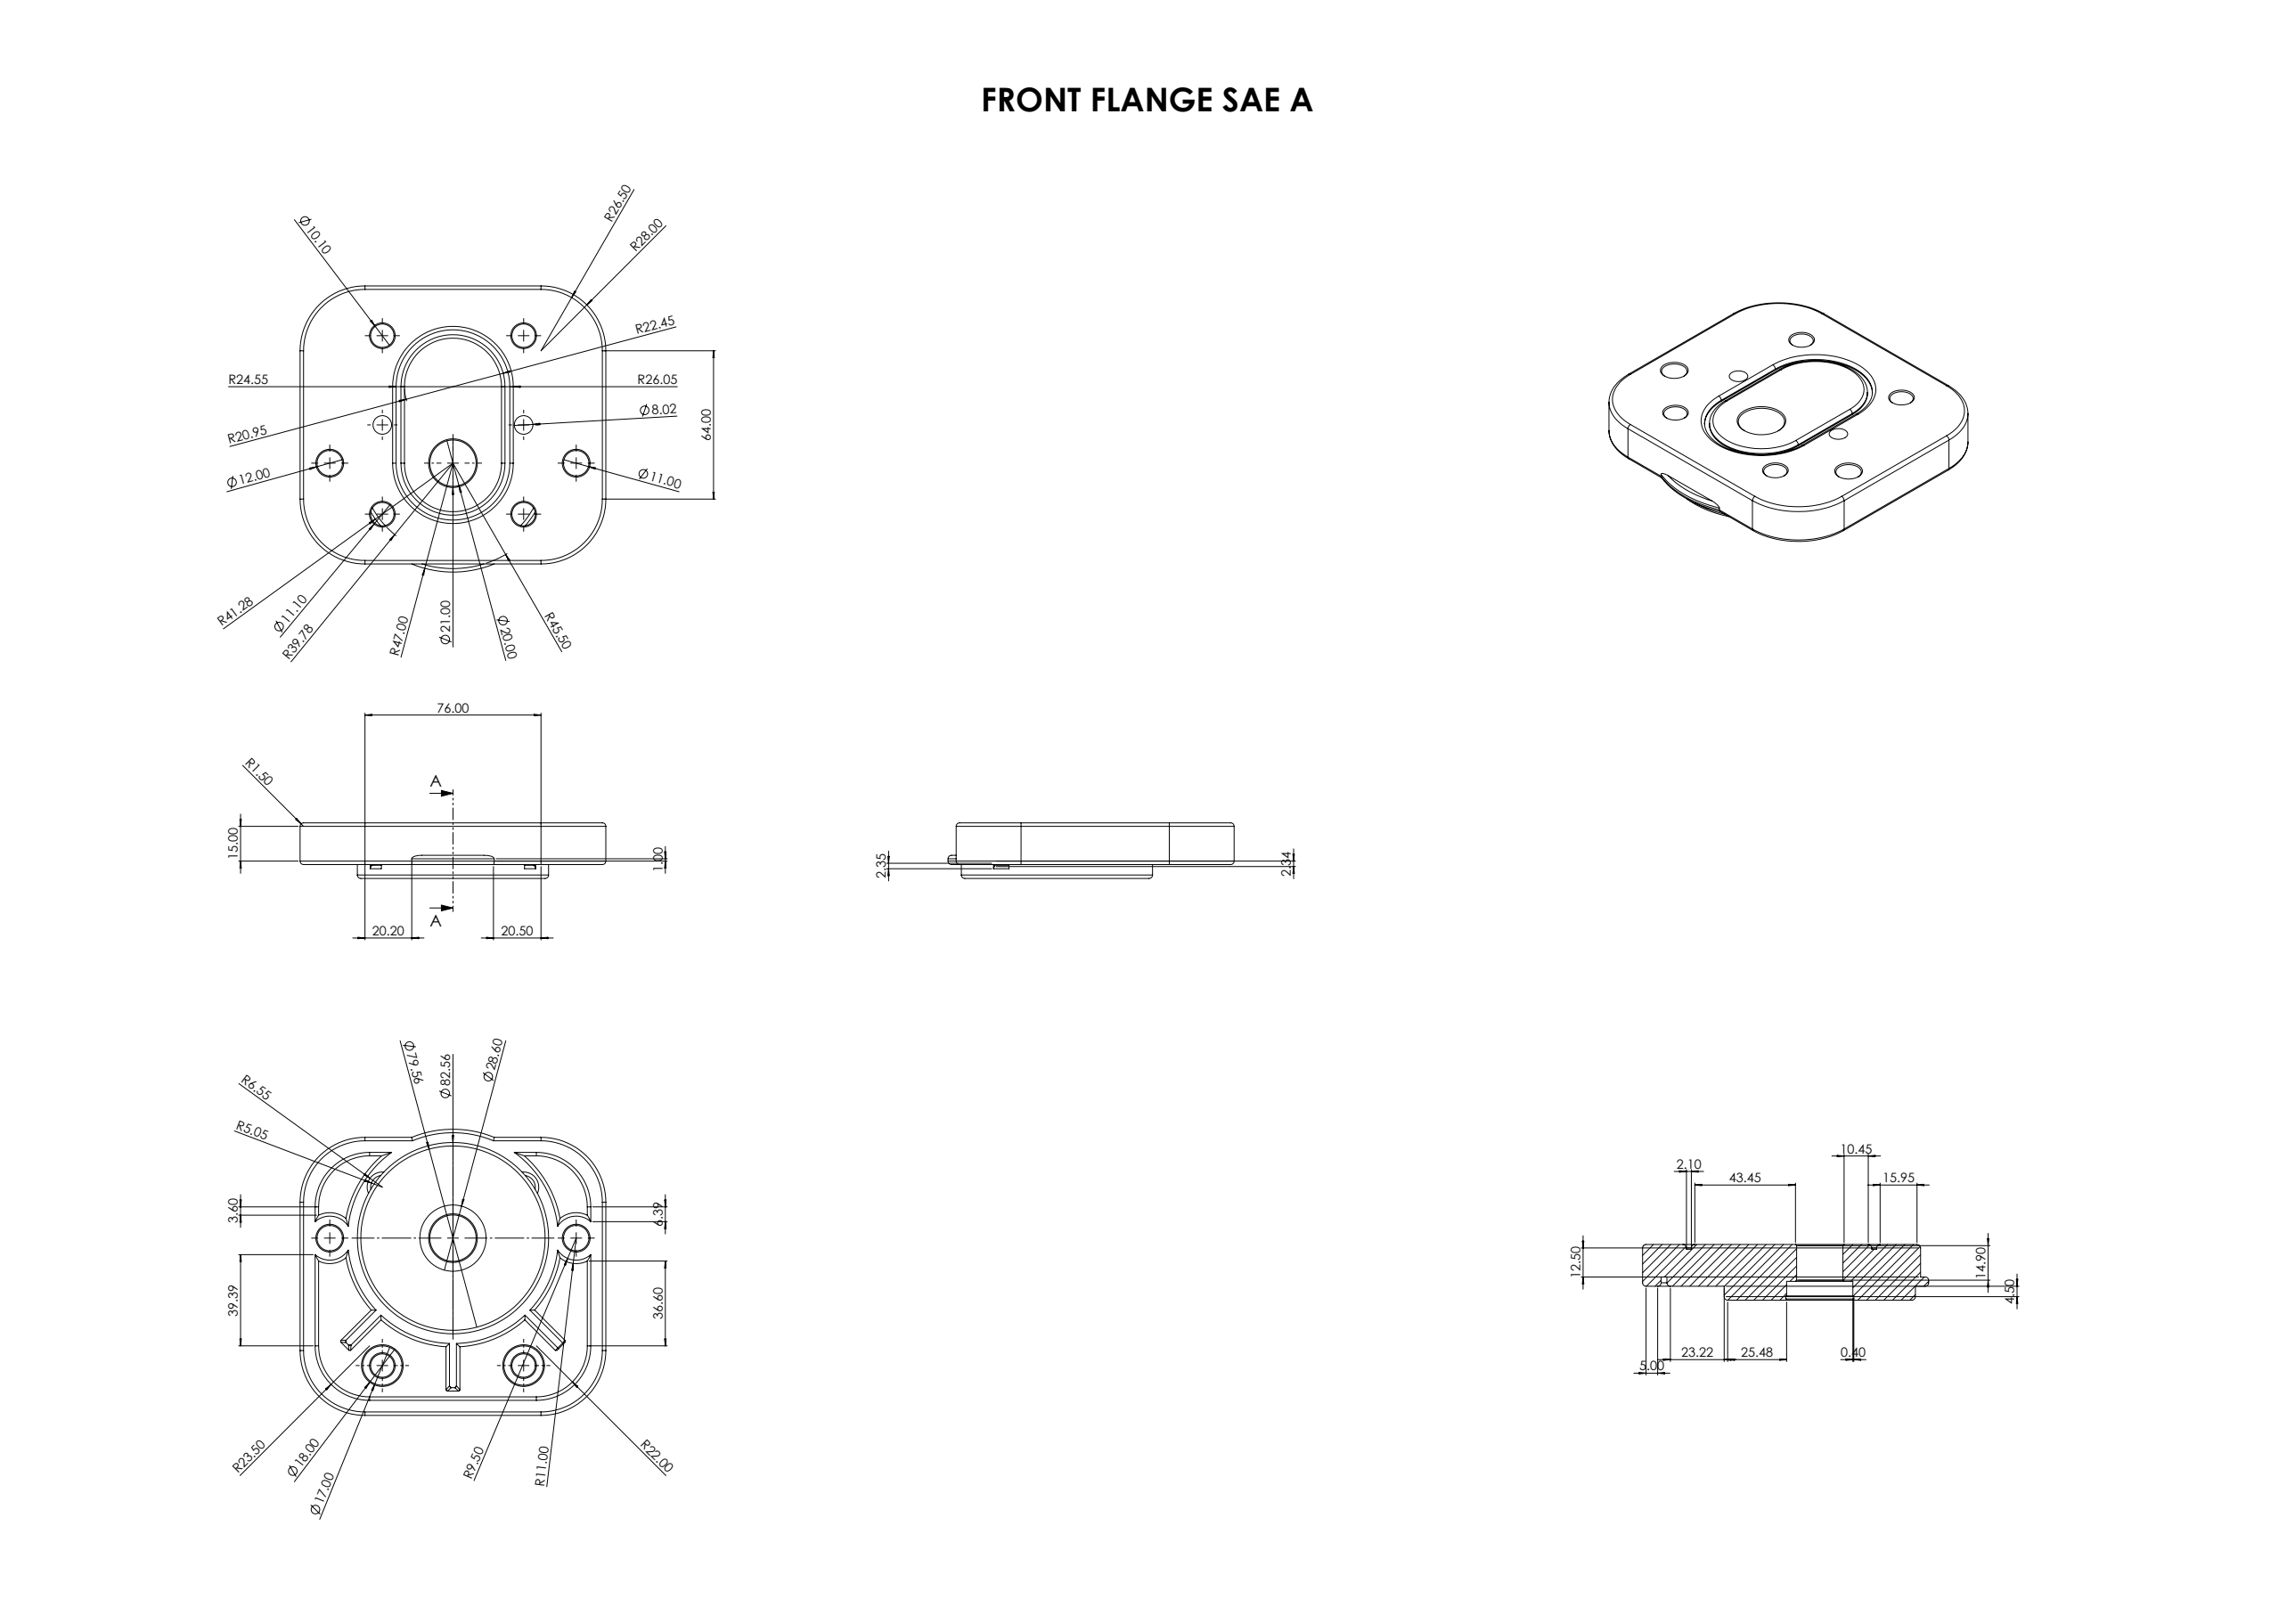
ISO-10303-21;
HEADER;
/* Generated by software containing ST-Developer
 * from STEP Tools, Inc. (www.steptools.com) 
 */

FILE_DESCRIPTION(
/* description */ (''),
/* implementation_level */ '2;1');

FILE_NAME(
/* name */ '01_Front_Flange_SAE_A.step',
/* time_stamp */ '2026-10-26T06:59:52-07:00',
/* author */ (''),
/* organization */ (''),
/* preprocessor_version */ 'ST-DEVELOPER v20.2',
/* originating_system */ 'Autodesk Translation Framework v15.15.0.0',
/* authorisation */ '');

FILE_SCHEMA (('AUTOMOTIVE_DESIGN { 1 0 10303 214 3 1 1 }'));
ENDSEC;

DATA;
#10=MECHANICAL_DESIGN_GEOMETRIC_PRESENTATION_REPRESENTATION('',(#164),#46395);
#136=SHAPE_REPRESENTATION_RELATIONSHIP('SRR','None',#46456,#150);
#150=ADVANCED_BREP_SHAPE_REPRESENTATION('',(#178),#46381);
#164=STYLED_ITEM('',(#46589),#178);
#178=MANIFOLD_SOLID_BREP('Body1',#24937);
#192=TOROIDAL_SURFACE('',#25235,45.5,1.5);
#193=TOROIDAL_SURFACE('',#25240,9.5,1.5);
#194=TOROIDAL_SURFACE('',#25242,45.5,1.5);
#195=TOROIDAL_SURFACE('',#25244,23.5,1.5);
#196=TOROIDAL_SURFACE('',#25255,45.5,1.5);
#197=TOROIDAL_SURFACE('',#25257,9.5,1.5);
#198=TOROIDAL_SURFACE('',#25259,23.5,1.5);
#199=TOROIDAL_SURFACE('',#25270,45.5,1.5);
#200=TOROIDAL_SURFACE('',#25271,45.5,1.5);
#201=TOROIDAL_SURFACE('',#25275,9.5,1.5);
#202=TOROIDAL_SURFACE('',#25281,9.5,1.5);
#203=TOROIDAL_SURFACE('',#25283,45.5,1.5);
#204=TOROIDAL_SURFACE('',#25285,23.5,1.5);
#205=TOROIDAL_SURFACE('',#25290,23.5,1.5);
#206=TOROIDAL_SURFACE('',#25308,26.5,1.5);
#207=TOROIDAL_SURFACE('',#25313,26.5,1.5);
#208=TOROIDAL_SURFACE('',#25318,26.5,1.5);
#209=TOROIDAL_SURFACE('',#25322,26.5,1.5);
#210=TOROIDAL_SURFACE('',#25338,45.5,1.5);
#211=TOROIDAL_SURFACE('',#25341,45.5,1.5);
#212=TOROIDAL_SURFACE('',#25348,26.5,1.5);
#213=TOROIDAL_SURFACE('',#25353,26.5,1.5);
#214=TOROIDAL_SURFACE('',#25357,26.5,1.5);
#215=TOROIDAL_SURFACE('',#25361,26.5,1.5);
#216=TOROIDAL_SURFACE('',#25365,39.78,1.5);
#217=TOROIDAL_SURFACE('',#25376,6.55,1.5);
#218=TOROIDAL_SURFACE('',#25377,39.78,1.5);
#219=TOROIDAL_SURFACE('',#25380,6.55,1.5);
#220=TOROIDAL_SURFACE('',#25381,39.78,1.5);
#221=TOROIDAL_SURFACE('',#25387,26.05,1.5);
#222=TOROIDAL_SURFACE('',#25392,26.05,1.5);
#223=TOROIDAL_SURFACE('',#25400,20.95,1.5);
#224=TOROIDAL_SURFACE('',#25405,20.95,1.5);
#235=B_SPLINE_CURVE_WITH_KNOTS('',3,(#33538,#33539,#33540,#33541,#33542,
#33543,#33544,#33545,#33546,#33547,#33548,#33549,#33550,#33551,#33552,#33553,
#33554,#33555,#33556,#33557,#33558,#33559,#33560,#33561,#33562,#33563,#33564,
#33565,#33566,#33567,#33568,#33569,#33570,#33571,#33572,#33573,#33574,#33575,
#33576,#33577,#33578,#33579,#33580,#33581,#33582,#33583,#33584,#33585,#33586,
#33587,#33588,#33589,#33590,#33591,#33592),.UNSPECIFIED.,.F.,.F.,(4,3,3,
3,3,3,3,3,3,3,3,3,3,3,3,3,3,3,4),(0.,0.0454718630237578,0.0931953780608733,
0.144039899823244,0.200168007589431,0.270586701890984,0.345292422598273,
0.401891619290293,0.45296463277568,0.503347839954974,0.552485563142507,
0.605298848839098,0.665634056697671,0.749225542523253,0.81191915689244,
0.864445081090996,0.913828865900519,0.959856605633726,1.),.UNSPECIFIED.);
#236=B_SPLINE_CURVE_WITH_KNOTS('',3,(#33594,#33595,#33596,#33597),
 .UNSPECIFIED.,.F.,.F.,(4,4),(0.,1.),.UNSPECIFIED.);
#237=B_SPLINE_CURVE_WITH_KNOTS('',3,(#33599,#33600,#33601,#33602,#33603,
#33604,#33605,#33606,#33607,#33608,#33609,#33610,#33611,#33612,#33613,#33614,
#33615,#33616,#33617,#33618,#33619,#33620,#33621,#33622,#33623,#33624,#33625,
#33626,#33627,#33628,#33629,#33630,#33631,#33632,#33633,#33634,#33635,#33636,
#33637,#33638,#33639,#33640,#33641,#33642,#33643,#33644,#33645,#33646,#33647,
#33648,#33649,#33650,#33651,#33652,#33653),.UNSPECIFIED.,.F.,.F.,(4,3,3,
3,3,3,3,3,3,3,3,3,3,3,3,3,3,3,4),(0.,0.0454743571758902,0.0932006890496271,
0.144048574957132,0.200181673047708,0.270614812390332,0.345307027643268,
0.401906381576284,0.452980318796508,0.503379519506553,0.552517196305264,
0.605331277143632,0.665671120969931,0.749253340727448,0.811940005545586,
0.864461351673364,0.913841478931635,0.959866376898225,1.),.UNSPECIFIED.);
#238=B_SPLINE_CURVE_WITH_KNOTS('',3,(#33680,#33681,#33682,#33683,#33684,
#33685),.UNSPECIFIED.,.F.,.F.,(4,1,1,4),(-1.75610615531805,-1.00348923161032,
-0.501744615805158,5.55111512312578E-16),.UNSPECIFIED.);
#239=B_SPLINE_CURVE_WITH_KNOTS('',3,(#33688,#33689,#33690,#33691,#33692,
#33693),.UNSPECIFIED.,.F.,.F.,(4,1,1,4),(-5.55111512312578E-16,0.501744615805158,
1.00348923161032,1.75610615531805),.UNSPECIFIED.);
#240=B_SPLINE_CURVE_WITH_KNOTS('',3,(#33804,#33805,#33806,#33807,#33808,
#33809,#33810),.UNSPECIFIED.,.F.,.F.,(4,1,1,1,4),(-1.75610615531805,-1.25436153951289,
-0.752616923707736,-0.501744615805158,1.11022302462516E-16),
 .UNSPECIFIED.);
#241=B_SPLINE_CURVE_WITH_KNOTS('',3,(#33811,#33812,#33813,#33814,#33815,
#33816,#33817,#33818,#33819,#33820,#33821,#33822,#33823,#33824,#33825,#33826,
#33827,#33828,#33829,#33830,#33831,#33832,#33833,#33834,#33835,#33836,#33837,
#33838,#33839,#33840,#33841,#33842,#33843,#33844,#33845,#33846,#33847,#33848,
#33849,#33850,#33851,#33852,#33853,#33854,#33855,#33856,#33857,#33858,#33859,
#33860,#33861,#33862,#33863,#33864,#33865),.UNSPECIFIED.,.F.,.F.,(4,3,3,
3,3,3,3,3,3,3,3,3,3,3,3,3,3,3,4),(0.,0.0454718630243312,0.0931953780626333,
0.144039899827111,0.200168007593285,0.270586701897688,0.345292422601244,
0.401891619293199,0.452964632777224,0.503347839955881,0.552485563143915,
0.605298848838407,0.665634056695417,0.749225542521563,0.811919156891172,
0.864445081089317,0.913828865898997,0.959856605632299,1.),.UNSPECIFIED.);
#242=B_SPLINE_CURVE_WITH_KNOTS('',3,(#33895,#33896,#33897,#33898),
 .UNSPECIFIED.,.F.,.F.,(4,4),(0.,1.),.UNSPECIFIED.);
#243=B_SPLINE_CURVE_WITH_KNOTS('',3,(#33899,#33900,#33901,#33902,#33903,
#33904,#33905,#33906,#33907,#33908,#33909,#33910,#33911,#33912,#33913,#33914,
#33915,#33916,#33917,#33918,#33919,#33920,#33921,#33922,#33923,#33924,#33925,
#33926,#33927,#33928,#33929,#33930,#33931,#33932,#33933,#33934,#33935,#33936,
#33937,#33938,#33939,#33940,#33941,#33942,#33943,#33944,#33945,#33946,#33947,
#33948,#33949,#33950,#33951,#33952,#33953),.UNSPECIFIED.,.F.,.F.,(4,3,3,
3,3,3,3,3,3,3,3,3,3,3,3,3,3,3,4),(0.,0.0454743571758495,0.0932006890494206,
0.144048574957566,0.200181673048685,0.270614812390706,0.345307027641822,
0.401906381575635,0.452980318795634,0.503379519504597,0.552517196303257,
0.605331277141522,0.665671120968433,0.749253340726325,0.811940005544743,
0.864461351672607,0.913841478930594,0.959866376897371,1.),.UNSPECIFIED.);
#244=B_SPLINE_CURVE_WITH_KNOTS('',3,(#33984,#33985,#33986,#33987,#33988,
#33989,#33990),.UNSPECIFIED.,.F.,.F.,(4,1,1,1,4),(-1.11022302462516E-16,
0.501744615805158,0.752616923707736,1.25436153951289,1.75610615531805),
 .UNSPECIFIED.);
#245=B_SPLINE_CURVE_WITH_KNOTS('',3,(#33998,#33999,#34000,#34001,#34002,
#34003,#34004,#34005,#34006,#34007,#34008,#34009,#34010,#34011),
 .UNSPECIFIED.,.F.,.F.,(4,2,2,2,2,2,4),(0.2830029806958,0.32673657269417,
0.376100941370913,0.440377410457652,0.50187293467793,0.56600596139079,0.566744275786352),
 .UNSPECIFIED.);
#246=B_SPLINE_CURVE_WITH_KNOTS('',3,(#34035,#34036,#34037,#34038,#34039,
#34040),.UNSPECIFIED.,.F.,.F.,(4,2,4),(0.457345926229208,0.511458202087047,
0.555227226239397),.UNSPECIFIED.);
#247=B_SPLINE_CURVE_WITH_KNOTS('',3,(#34044,#34045,#34046,#34047,#34048,
#34049),.UNSPECIFIED.,.F.,.F.,(4,2,4),(0.,0.0542493992714901,0.0984920623079337),
 .UNSPECIFIED.);
#248=B_SPLINE_CURVE_WITH_KNOTS('',3,(#34058,#34059,#34060,#34061,#34062,
#34063,#34064,#34065),.UNSPECIFIED.,.F.,.F.,(4,2,2,4),(0.,0.0729822624604683,
0.159547666524593,0.160512003570787),.UNSPECIFIED.);
#249=B_SPLINE_CURVE_WITH_KNOTS('',3,(#34071,#34072,#34073,#34074,#34075,
#34076,#34077,#34078),.UNSPECIFIED.,.F.,.F.,(4,2,2,4),(0.883241961717341,
0.890937005468247,0.9697019851369,1.04402990736473),.UNSPECIFIED.);
#250=B_SPLINE_CURVE_WITH_KNOTS('',3,(#34083,#34084,#34085,#34086,#34087,
#34088),.UNSPECIFIED.,.F.,.F.,(4,2,4),(-0.0984920602555225,-0.0542493992714899,
0.),.UNSPECIFIED.);
#251=B_SPLINE_CURVE_WITH_KNOTS('',3,(#34092,#34093,#34094,#34095,#34096,
#34097),.UNSPECIFIED.,.F.,.F.,(4,2,4),(0.359464626219636,0.403233650371369,
0.457345926229208),.UNSPECIFIED.);
#252=B_SPLINE_CURVE_WITH_KNOTS('',3,(#34106,#34107,#34108,#34109,#34110,
#34111,#34112,#34113),.UNSPECIFIED.,.F.,.F.,(4,2,2,4),(0.883254863276601,
0.890921572363312,0.969698219486375,1.04404196291709),.UNSPECIFIED.);
#253=B_SPLINE_CURVE_WITH_KNOTS('',3,(#34117,#34118,#34119,#34120,#34121,
#34122,#34123,#34124),.UNSPECIFIED.,.F.,.F.,(4,2,2,4),(0.,0.0729893210250683,
0.159554275962458,0.160511436887519),.UNSPECIFIED.);
#254=B_SPLINE_CURVE_WITH_KNOTS('',3,(#34130,#34131,#34132,#34133,#34134,
#34135),.UNSPECIFIED.,.F.,.F.,(4,2,4),(0.457345926229207,0.511458202087047,
0.555227226239396),.UNSPECIFIED.);
#255=B_SPLINE_CURVE_WITH_KNOTS('',3,(#34137,#34138,#34139,#34140,#34141,
#34142),.UNSPECIFIED.,.F.,.F.,(4,2,4),(0.,0.0542493992714896,0.0984920622777539),
 .UNSPECIFIED.);
#256=B_SPLINE_CURVE_WITH_KNOTS('',3,(#34146,#34147,#34148,#34149,#34150,
#34151),.UNSPECIFIED.,.F.,.F.,(4,2,4),(-0.0984920602555227,-0.0542493992714901,
0.),.UNSPECIFIED.);
#257=B_SPLINE_CURVE_WITH_KNOTS('',3,(#34153,#34154,#34155,#34156,#34157,
#34158),.UNSPECIFIED.,.F.,.F.,(4,2,4),(0.359464626219636,0.403233650371367,
0.457345926229207),.UNSPECIFIED.);
#258=B_SPLINE_CURVE_WITH_KNOTS('',3,(#34250,#34251,#34252,#34253,#34254,
#34255,#34256,#34257,#34258,#34259,#34260,#34261,#34262,#34263,#34264,#34265,
#34266,#34267,#34268,#34269,#34270,#34271,#34272,#34273,#34274,#34275,#34276,
#34277,#34278,#34279,#34280,#34281,#34282,#34283,#34284,#34285,#34286,#34287,
#34288,#34289,#34290,#34291,#34292,#34293,#34294,#34295,#34296,#34297,#34298,
#34299,#34300,#34301,#34302,#34303,#34304),.UNSPECIFIED.,.F.,.F.,(4,3,3,
3,3,3,3,3,3,3,3,3,3,3,3,3,3,3,4),(0.,0.0454718630236453,0.0931953780618335,
0.144039899826865,0.200168007592162,0.270586701896513,0.345292422605783,
0.401891619297809,0.452964632782272,0.503347839964507,0.552485563152053,
0.605298848849878,0.665634056712773,0.74922554253458,0.811919156900935,
0.864445081098314,0.913828865908445,0.959856605641832,1.),.UNSPECIFIED.);
#259=B_SPLINE_CURVE_WITH_KNOTS('',3,(#34306,#34307,#34308,#34309),
 .UNSPECIFIED.,.F.,.F.,(4,4),(0.,1.),.UNSPECIFIED.);
#260=B_SPLINE_CURVE_WITH_KNOTS('',3,(#34310,#34311,#34312,#34313,#34314,
#34315,#34316,#34317,#34318,#34319,#34320,#34321,#34322,#34323,#34324,#34325,
#34326,#34327,#34328,#34329,#34330,#34331,#34332,#34333,#34334,#34335,#34336,
#34337,#34338,#34339,#34340,#34341,#34342,#34343,#34344,#34345,#34346,#34347,
#34348,#34349,#34350,#34351,#34352,#34353,#34354,#34355,#34356,#34357,#34358,
#34359,#34360,#34361,#34362,#34363,#34364),.UNSPECIFIED.,.F.,.F.,(4,3,3,
3,3,3,3,3,3,3,3,3,3,3,3,3,3,3,4),(0.,0.0454743571759648,0.0932006890496545,
0.144048574957612,0.200181673048621,0.270614812391917,0.345307027644055,
0.401906381576845,0.452980318797118,0.503379519507497,0.552517196306345,
0.605331277144942,0.665671120971507,0.74925334072863,0.811940005546473,
0.864461351674218,0.91384147893233,0.959866376898877,1.),.UNSPECIFIED.);
#261=B_SPLINE_CURVE_WITH_KNOTS('',3,(#34390,#34391,#34392,#34393,#34394,
#34395),.UNSPECIFIED.,.F.,.F.,(4,1,1,4),(-1.75610615531806,-1.00348923161031,
-0.501744615805142,2.47024622979097E-14),.UNSPECIFIED.);
#262=B_SPLINE_CURVE_WITH_KNOTS('',3,(#34398,#34399,#34400,#34401,#34402,
#34403),.UNSPECIFIED.,.F.,.F.,(4,1,1,4),(-2.47024622979097E-14,0.501744615805142,
1.00348923161031,1.75610615531806),.UNSPECIFIED.);
#263=B_SPLINE_CURVE_WITH_KNOTS('',3,(#34414,#34415,#34416,#34417,#34418,
#34419),.UNSPECIFIED.,.F.,.F.,(4,1,1,4),(-1.75610615531805,-1.00348923161031,
-0.501744615805157,-5.27355936696957E-16),.UNSPECIFIED.);
#264=B_SPLINE_CURVE_WITH_KNOTS('',3,(#34420,#34421,#34422,#34423,#34424,
#34425,#34426,#34427,#34428,#34429,#34430,#34431,#34432,#34433,#34434,#34435,
#34436,#34437,#34438,#34439,#34440,#34441,#34442,#34443,#34444,#34445,#34446,
#34447,#34448,#34449,#34450,#34451,#34452,#34453,#34454,#34455,#34456,#34457,
#34458,#34459,#34460,#34461,#34462,#34463,#34464,#34465,#34466,#34467,#34468,
#34469,#34470,#34471,#34472,#34473,#34474),.UNSPECIFIED.,.F.,.F.,(4,3,3,
3,3,3,3,3,3,3,3,3,3,3,3,3,3,3,4),(0.,0.0454718630243914,0.0931953780626216,
0.14403989982724,0.200168007593373,0.270586701897748,0.345292422601248,
0.401891619293078,0.452964632777054,0.50334783995564,0.552485563143574,
0.605298848838025,0.665634056695,0.74922554252125,0.811919156890937,0.864445081089107,
0.91382886589878,0.959856605632085,1.),.UNSPECIFIED.);
#265=B_SPLINE_CURVE_WITH_KNOTS('',3,(#34504,#34505,#34506,#34507),
 .UNSPECIFIED.,.F.,.F.,(4,4),(0.,1.),.UNSPECIFIED.);
#266=B_SPLINE_CURVE_WITH_KNOTS('',3,(#34508,#34509,#34510,#34511,#34512,
#34513,#34514,#34515,#34516,#34517,#34518,#34519,#34520,#34521,#34522,#34523,
#34524,#34525,#34526,#34527,#34528,#34529,#34530,#34531,#34532,#34533,#34534,
#34535,#34536,#34537,#34538,#34539,#34540,#34541,#34542,#34543,#34544,#34545,
#34546,#34547,#34548,#34549,#34550,#34551,#34552,#34553,#34554,#34555,#34556,
#34557,#34558,#34559,#34560,#34561,#34562),.UNSPECIFIED.,.F.,.F.,(4,3,3,
3,3,3,3,3,3,3,3,3,3,3,3,3,3,3,4),(0.,0.0454743571761675,0.0932006890500933,
0.144048574956671,0.200181673048282,0.270614812391009,0.345307027645443,
0.401906381578876,0.452980318799016,0.503379519512151,0.552517196310239,
0.605331277149278,0.665671120975839,0.749253340731879,0.81194000554891,
0.864461351676132,0.91384147893387,0.959866376900601,1.),.UNSPECIFIED.);
#267=B_SPLINE_CURVE_WITH_KNOTS('',3,(#34589,#34590,#34591,#34592,#34593,
#34594),.UNSPECIFIED.,.F.,.F.,(4,1,1,4),(5.27355936696957E-16,0.501744615805157,
1.00348923161031,1.75610615531805),.UNSPECIFIED.);
#268=B_SPLINE_CURVE_WITH_KNOTS('',3,(#34602,#34603,#34604,#34605,#34606,
#34607,#34608,#34609,#34610,#34611,#34612,#34613,#34614,#34615),
 .UNSPECIFIED.,.F.,.F.,(4,2,2,2,2,2,4),(-0.566727656910624,-0.565965930395602,
-0.501954114034259,-0.440929548119714,-0.376258061364955,-0.326742970835578,
-0.282982965197809),.UNSPECIFIED.);
#269=B_SPLINE_CURVE_WITH_KNOTS('',3,(#34659,#34660,#34661,#34662,#34663,
#34664,#34665,#34666,#34667,#34668,#34669,#34670),.UNSPECIFIED.,.F.,.F.,
(4,2,2,2,2,4),(0.,0.0177298768866499,0.0386480203638908,0.106699501354674,
0.29072652917135,0.474753556988026),.UNSPECIFIED.);
#270=B_SPLINE_CURVE_WITH_KNOTS('',3,(#34674,#34675,#34676,#34677,#34678,
#34679,#34680,#34681,#34682,#34683,#34684,#34685),.UNSPECIFIED.,.F.,.F.,
(4,2,2,2,2,4),(1.80681462537756,1.99084165319423,2.17486868101091,2.24292016200169,
2.26383830547893,2.28156818236558),.UNSPECIFIED.);
#271=B_SPLINE_CURVE_WITH_KNOTS('',3,(#34695,#34696,#34697,#34698,#34699,
#34700,#34701,#34702,#34703,#34704,#34705,#34706,#34707,#34708),
 .UNSPECIFIED.,.F.,.F.,(4,2,2,2,2,2,4),(-1.39612360577563,-1.39460700772923,
-1.17311194871629,-0.972537848487119,-0.846807900198276,-0.765057233826425,
-0.697303504183967),.UNSPECIFIED.);
#272=B_SPLINE_CURVE_WITH_KNOTS('',3,(#34711,#34712,#34713,#34714,#34715,
#34716,#34717,#34718,#34719,#34720,#34721,#34722,#34723,#34724),
 .UNSPECIFIED.,.F.,.F.,(4,2,2,2,2,2,4),(-0.00127041341091992,0.,0.142293631997042,
0.26745747621236,0.346088913132952,0.397847011808156,0.440929147841825),
 .UNSPECIFIED.);
#273=B_SPLINE_CURVE_WITH_KNOTS('',3,(#34727,#34728,#34729,#34730,#34731,
#34732,#34733,#34734,#34735,#34736,#34737,#34738,#34739,#34740),
 .UNSPECIFIED.,.F.,.F.,(4,2,2,2,2,2,4),(-1.41597302520629,-1.41418889589625,
-1.0666111176201,-0.892135751403682,-0.801536275589833,-0.748843387075389,
-0.707094447966972),.UNSPECIFIED.);
#274=B_SPLINE_CURVE_WITH_KNOTS('',3,(#34768,#34769,#34770,#34771,#34772,
#34773,#34774,#34775,#34776,#34777,#34778,#34779,#34780,#34781),
 .UNSPECIFIED.,.F.,.F.,(4,2,2,2,2,2,4),(-1.39362312416001,-1.39199898884262,
-1.17364167365164,-0.971197013124251,-0.845224951582453,-0.76357754542349,
-0.695999491978471),.UNSPECIFIED.);
#275=B_SPLINE_CURVE_WITH_KNOTS('',3,(#34784,#34785,#34786,#34787,#34788,
#34789,#34790,#34791,#34792,#34793,#34794,#34795,#34796,#34797),
 .UNSPECIFIED.,.F.,.F.,(4,2,2,2,2,2,4),(-0.00178412931182033,0.,0.347577778842949,
0.522053145574294,0.612652621655965,0.665345510326134,0.707094449558532),
 .UNSPECIFIED.);
#276=B_SPLINE_CURVE_WITH_KNOTS('',3,(#34800,#34801,#34802,#34803,#34804,
#34805,#34806,#34807,#34808,#34809,#34810,#34811,#34812,#34813),
 .UNSPECIFIED.,.F.,.F.,(4,2,2,2,2,2,4),(-0.883128709093834,-0.881858295682913,
-0.739564663685846,-0.614400819470615,-0.535769382550153,-0.484011283875034,
-0.440929147841436),.UNSPECIFIED.);
#277=B_SPLINE_CURVE_WITH_KNOTS('',3,(#34840,#34841,#34842,#34843,#34844,
#34845,#34846,#34847,#34848,#34849,#34850,#34851,#34852,#34853),
 .UNSPECIFIED.,.F.,.F.,(4,2,2,2,2,2,4),(0.237947781581816,0.295547529372161,
0.353697178748574,0.412988302648374,0.444419571172075,0.475895563163675,
0.476565408893143),.UNSPECIFIED.);
#278=B_SPLINE_CURVE_WITH_KNOTS('',3,(#34854,#34855,#34856,#34857,#34858,
#34859,#34860,#34861,#34862,#34863,#34864,#34865,#34866,#34867),
 .UNSPECIFIED.,.F.,.F.,(4,2,2,2,2,2,4),(-0.000669845729473591,0.,0.0314759919915142,
0.0629072605151251,0.122198384414748,0.180348033790988,0.237947781581162),
 .UNSPECIFIED.);
#279=B_SPLINE_CURVE_WITH_KNOTS('',3,(#34871,#34872,#34873,#34874,#34875,
#34876,#34877,#34878,#34879,#34880,#34881,#34882,#34883,#34884),
 .UNSPECIFIED.,.F.,.F.,(4,2,2,2,2,2,4),(-0.000737243235122344,0.,0.0641388256771107,
0.1256562494953,0.189914332907335,0.239271567314492,0.283003897177937),
 .UNSPECIFIED.);
#280=B_SPLINE_CURVE_WITH_KNOTS('',3,(#34891,#34892,#34893,#34894,#34895,
#34896,#34897,#34898,#34899,#34900,#34901,#34902,#34903,#34904),
 .UNSPECIFIED.,.F.,.F.,(4,2,2,2,2,2,4),(0.440929147841474,0.484011283875067,
0.53576938255019,0.614400819470681,0.739564663685834,0.881858295682709,
0.883128709093627),.UNSPECIFIED.);
#281=B_SPLINE_CURVE_WITH_KNOTS('',3,(#34907,#34908,#34909,#34910,#34911,
#34912,#34913,#34914,#34915,#34916,#34917,#34918,#34919,#34920),
 .UNSPECIFIED.,.F.,.F.,(4,2,2,2,2,2,4),(-0.00151659805374153,0.,0.221495058999754,
0.422069157956912,0.547799105448391,0.629549771301697,0.697303500514436),
 .UNSPECIFIED.);
#282=B_SPLINE_CURVE_WITH_KNOTS('',3,(#34932,#34933,#34934,#34935,#34936,
#34937,#34938,#34939,#34940,#34941,#34942,#34943,#34944,#34945),
 .UNSPECIFIED.,.F.,.F.,(4,2,2,2,2,2,4),(-0.00127041341147968,0.,0.142293632019536,
0.267457476256502,0.346088913190727,0.397847011874902,0.44092914791602),
 .UNSPECIFIED.);
#283=B_SPLINE_CURVE_WITH_KNOTS('',3,(#34948,#34949,#34950,#34951,#34952,
#34953,#34954,#34955,#34956,#34957,#34958,#34959,#34960,#34961),
 .UNSPECIFIED.,.F.,.F.,(4,2,2,2,2,2,4),(-1.39612359503373,-1.39460699698273,
-1.17311193853035,-0.972537840238686,-0.846807893164431,-0.765057227582403,
-0.697303498594505),.UNSPECIFIED.);
#284=B_SPLINE_CURVE_WITH_KNOTS('',3,(#34965,#34966,#34967,#34968,#34969,
#34970,#34971,#34972,#34973,#34974,#34975,#34976,#34977,#34978),
 .UNSPECIFIED.,.F.,.F.,(4,2,2,2,2,2,4),(0.283003897184326,0.326736227048831,
0.37609346145714,0.440351544870681,0.501868968690292,0.566007794368658,
0.566745037603787),.UNSPECIFIED.);
#285=B_SPLINE_CURVE_WITH_KNOTS('',3,(#35089,#35090,#35091,#35092,#35093,
#35094,#35095,#35096,#35097,#35098,#35099,#35100,#35101,#35102),
 .UNSPECIFIED.,.F.,.F.,(4,2,2,2,2,2,4),(-0.000738314395613078,0.,0.0641330267183371,
0.125628550943858,0.189905020036076,0.23926938871703,0.283002980719128),
 .UNSPECIFIED.);
#286=B_SPLINE_CURVE_WITH_KNOTS('',3,(#35105,#35106,#35107,#35108,#35109,
#35110,#35111,#35112,#35113,#35114,#35115,#35116,#35117,#35118),
 .UNSPECIFIED.,.F.,.F.,(4,2,2,2,2,2,4),(-0.000761726515024963,0.,0.0640118163614976,
0.125036382276213,0.189707869031154,0.239222959560681,0.282982965198561),
 .UNSPECIFIED.);
#287=B_SPLINE_CURVE_WITH_KNOTS('',3,(#35161,#35162,#35163,#35164,#35165,
#35166,#35167,#35168),.UNSPECIFIED.,.F.,.F.,(4,2,2,4),(0.9079700629405,
0.928682763365301,1.00209186414222,1.07647666313639),.UNSPECIFIED.);
#288=B_SPLINE_CURVE_WITH_KNOTS('',3,(#35169,#35170,#35171,#35172,#35173,
#35174),.UNSPECIFIED.,.F.,.F.,(4,2,4),(0.,0.0943434934286175,0.17124459577731),
 .UNSPECIFIED.);
#289=B_SPLINE_CURVE_WITH_KNOTS('',3,(#35176,#35177,#35178,#35179,#35180,
#35181,#35182,#35183),.UNSPECIFIED.,.F.,.F.,(4,2,2,4),(0.907970062940467,
0.928682763365269,1.00209186414218,1.07647666313636),.UNSPECIFIED.);
#290=B_SPLINE_CURVE_WITH_KNOTS('',3,(#35185,#35186,#35187,#35188,#35189,
#35190),.UNSPECIFIED.,.F.,.F.,(4,2,4),(0.,0.0943434934286164,0.171244595777307),
 .UNSPECIFIED.);
#390=B_SPLINE_SURFACE_WITH_KNOTS('',3,3,((#33512,#33513,#33514,#33515,#33516,
#33517),(#33518,#33519,#33520,#33521,#33522,#33523),(#33524,#33525,#33526,
#33527,#33528,#33529),(#33530,#33531,#33532,#33533,#33534,#33535)),
 .UNSPECIFIED.,.F.,.F.,.F.,(4,4),(4,1,1,4),(0.,1.),(0.,0.571428571428571,
0.857142857142857,1.),.UNSPECIFIED.);
#391=B_SPLINE_SURFACE_WITH_KNOTS('',3,3,((#33655,#33656,#33657,#33658,#33659,
#33660),(#33661,#33662,#33663,#33664,#33665,#33666),(#33667,#33668,#33669,
#33670,#33671,#33672),(#33673,#33674,#33675,#33676,#33677,#33678)),
 .UNSPECIFIED.,.F.,.F.,.F.,(4,4),(4,1,1,4),(0.,1.),(-1.75610615531805,-1.00348923161032,
-0.501744615805158,5.55111512312578E-16),.UNSPECIFIED.);
#392=B_SPLINE_SURFACE_WITH_KNOTS('',3,3,((#33870,#33871,#33872,#33873,#33874,
#33875),(#33876,#33877,#33878,#33879,#33880,#33881),(#33882,#33883,#33884,
#33885,#33886,#33887),(#33888,#33889,#33890,#33891,#33892,#33893)),
 .UNSPECIFIED.,.F.,.F.,.F.,(4,4),(4,1,1,4),(0.,1.),(0.,0.571428571428571,
0.857142857142857,1.),.UNSPECIFIED.);
#393=B_SPLINE_SURFACE_WITH_KNOTS('',3,3,((#33954,#33955,#33956,#33957,#33958,
#33959,#33960),(#33961,#33962,#33963,#33964,#33965,#33966,#33967),(#33968,
#33969,#33970,#33971,#33972,#33973,#33974),(#33975,#33976,#33977,#33978,
#33979,#33980,#33981)),.UNSPECIFIED.,.F.,.F.,.F.,(4,4),(4,1,1,1,4),(0.,
1.),(-1.75610615531805,-1.25436153951289,-0.752616923707736,-0.501744615805158,
1.11022302462516E-16),.UNSPECIFIED.);
#394=B_SPLINE_SURFACE_WITH_KNOTS('',3,3,((#34225,#34226,#34227,#34228,#34229,
#34230),(#34231,#34232,#34233,#34234,#34235,#34236),(#34237,#34238,#34239,
#34240,#34241,#34242),(#34243,#34244,#34245,#34246,#34247,#34248)),
 .UNSPECIFIED.,.F.,.F.,.F.,(4,4),(4,1,1,4),(0.,1.),(0.,0.571428571428571,
0.857142857142857,1.),.UNSPECIFIED.);
#395=B_SPLINE_SURFACE_WITH_KNOTS('',3,3,((#34365,#34366,#34367,#34368,#34369,
#34370),(#34371,#34372,#34373,#34374,#34375,#34376),(#34377,#34378,#34379,
#34380,#34381,#34382),(#34383,#34384,#34385,#34386,#34387,#34388)),
 .UNSPECIFIED.,.F.,.F.,.F.,(4,4),(4,1,1,4),(0.,1.),(-1.75610615531806,-1.00348923161031,
-0.501744615805142,2.47024622979097E-14),.UNSPECIFIED.);
#396=B_SPLINE_SURFACE_WITH_KNOTS('',3,3,((#34479,#34480,#34481,#34482,#34483,
#34484),(#34485,#34486,#34487,#34488,#34489,#34490),(#34491,#34492,#34493,
#34494,#34495,#34496),(#34497,#34498,#34499,#34500,#34501,#34502)),
 .UNSPECIFIED.,.F.,.F.,.F.,(4,4),(4,1,1,4),(0.,1.),(0.,0.571428571428571,
0.857142857142857,1.),.UNSPECIFIED.);
#397=B_SPLINE_SURFACE_WITH_KNOTS('',3,3,((#34563,#34564,#34565,#34566,#34567,
#34568),(#34569,#34570,#34571,#34572,#34573,#34574),(#34575,#34576,#34577,
#34578,#34579,#34580),(#34581,#34582,#34583,#34584,#34585,#34586)),
 .UNSPECIFIED.,.F.,.F.,.F.,(4,4),(4,1,1,4),(0.,1.),(-1.75610615531805,-1.00348923161031,
-0.501744615805157,-5.27355936696957E-16),.UNSPECIFIED.);
#400=CYLINDRICAL_SURFACE('',#25113,9.);
#401=CYLINDRICAL_SURFACE('',#25120,9.);
#402=CYLINDRICAL_SURFACE('',#25126,10.);
#403=CYLINDRICAL_SURFACE('',#25163,1.5);
#404=CYLINDRICAL_SURFACE('',#25166,1.5);
#405=CYLINDRICAL_SURFACE('',#25170,5.05);
#406=CYLINDRICAL_SURFACE('',#25174,5.05);
#407=CYLINDRICAL_SURFACE('',#25177,5.05);
#408=CYLINDRICAL_SURFACE('',#25183,5.05);
#409=CYLINDRICAL_SURFACE('',#25211,5.5);
#410=CYLINDRICAL_SURFACE('',#25215,5.5);
#411=CYLINDRICAL_SURFACE('',#25218,1.5);
#412=CYLINDRICAL_SURFACE('',#25221,1.5);
#413=CYLINDRICAL_SURFACE('',#25238,47.);
#414=CYLINDRICAL_SURFACE('',#25248,1.5);
#415=CYLINDRICAL_SURFACE('',#25249,1.5);
#416=CYLINDRICAL_SURFACE('',#25250,47.);
#417=CYLINDRICAL_SURFACE('',#25253,22.);
#418=CYLINDRICAL_SURFACE('',#25263,1.5);
#419=CYLINDRICAL_SURFACE('',#25264,1.5);
#420=CYLINDRICAL_SURFACE('',#25265,11.);
#421=CYLINDRICAL_SURFACE('',#25268,22.);
#422=CYLINDRICAL_SURFACE('',#25273,47.);
#423=CYLINDRICAL_SURFACE('',#25277,11.);
#424=CYLINDRICAL_SURFACE('',#25279,1.5);
#425=CYLINDRICAL_SURFACE('',#25288,1.5);
#426=CYLINDRICAL_SURFACE('',#25293,1.5);
#427=CYLINDRICAL_SURFACE('',#25295,22.);
#428=CYLINDRICAL_SURFACE('',#25298,22.);
#429=CYLINDRICAL_SURFACE('',#25301,11.);
#430=CYLINDRICAL_SURFACE('',#25303,47.);
#431=CYLINDRICAL_SURFACE('',#25305,1.5);
#432=CYLINDRICAL_SURFACE('',#25311,1.5);
#433=CYLINDRICAL_SURFACE('',#25316,1.5);
#434=CYLINDRICAL_SURFACE('',#25321,1.5);
#435=CYLINDRICAL_SURFACE('',#25325,1.5);
#436=CYLINDRICAL_SURFACE('',#25326,28.);
#437=CYLINDRICAL_SURFACE('',#25329,28.);
#438=CYLINDRICAL_SURFACE('',#25332,28.);
#439=CYLINDRICAL_SURFACE('',#25334,1.5);
#440=CYLINDRICAL_SURFACE('',#25336,1.5);
#441=CYLINDRICAL_SURFACE('',#25340,1.5);
#442=CYLINDRICAL_SURFACE('',#25343,47.);
#443=CYLINDRICAL_SURFACE('',#25346,47.);
#444=CYLINDRICAL_SURFACE('',#25351,1.5);
#445=CYLINDRICAL_SURFACE('',#25355,1.5);
#446=CYLINDRICAL_SURFACE('',#25359,1.5);
#447=CYLINDRICAL_SURFACE('',#25364,1.5);
#448=CYLINDRICAL_SURFACE('',#25369,41.28);
#449=CYLINDRICAL_SURFACE('',#25374,1.5);
#450=CYLINDRICAL_SURFACE('',#25384,1.5);
#451=CYLINDRICAL_SURFACE('',#25390,1.5);
#452=CYLINDRICAL_SURFACE('',#25394,24.55);
#453=CYLINDRICAL_SURFACE('',#25397,1.5);
#454=CYLINDRICAL_SURFACE('',#25403,1.5);
#455=CYLINDRICAL_SURFACE('',#25407,22.45);
#456=CYLINDRICAL_SURFACE('',#25410,22.45);
#457=CYLINDRICAL_SURFACE('',#25413,24.55);
#458=CYLINDRICAL_SURFACE('',#25417,4.01);
#459=CYLINDRICAL_SURFACE('',#25420,4.01);
#460=CYLINDRICAL_SURFACE('',#25426,14.7);
#461=CYLINDRICAL_SURFACE('',#25430,14.3);
#462=CYLINDRICAL_SURFACE('',#25431,14.3);
#463=CYLINDRICAL_SURFACE('',#25433,47.);
#464=CYLINDRICAL_SURFACE('',#25435,11.);
#465=CYLINDRICAL_SURFACE('',#25444,28.);
#586=FACE_BOUND('',#3080,.T.);
#587=FACE_BOUND('',#3084,.T.);
#588=FACE_BOUND('',#3089,.T.);
#589=FACE_BOUND('',#3092,.T.);
#590=FACE_BOUND('',#3097,.T.);
#591=FACE_BOUND('',#3098,.T.);
#592=FACE_BOUND('',#3099,.T.);
#593=FACE_BOUND('',#3100,.T.);
#594=FACE_BOUND('',#3101,.T.);
#595=FACE_BOUND('',#3102,.T.);
#596=FACE_BOUND('',#3122,.T.);
#597=FACE_BOUND('',#3123,.T.);
#598=FACE_BOUND('',#3124,.T.);
#599=FACE_BOUND('',#3125,.T.);
#600=FACE_BOUND('',#3126,.T.);
#601=FACE_BOUND('',#3127,.T.);
#602=FACE_BOUND('',#3128,.T.);
#603=FACE_BOUND('',#3129,.T.);
#604=FACE_BOUND('',#3130,.T.);
#605=FACE_BOUND('',#3228,.T.);
#606=FACE_BOUND('',#3254,.T.);
#607=FACE_BOUND('',#3260,.T.);
#608=FACE_BOUND('',#3263,.T.);
#609=FACE_BOUND('',#3267,.T.);
#610=FACE_BOUND('',#3268,.T.);
#711=PLANE('',#25111);
#712=PLANE('',#25118);
#713=PLANE('',#25128);
#714=PLANE('',#25132);
#715=PLANE('',#25135);
#716=PLANE('',#25136);
#717=PLANE('',#25164);
#718=PLANE('',#25165);
#719=PLANE('',#25167);
#720=PLANE('',#25176);
#721=PLANE('',#25182);
#722=PLANE('',#25188);
#723=PLANE('',#25189);
#724=PLANE('',#25192);
#725=PLANE('',#25217);
#726=PLANE('',#25219);
#727=PLANE('',#25220);
#728=PLANE('',#25222);
#729=PLANE('',#25225);
#730=PLANE('',#25229);
#731=PLANE('',#25233);
#732=PLANE('',#25234);
#733=PLANE('',#25252);
#734=PLANE('',#25267);
#735=PLANE('',#25294);
#736=PLANE('',#25297);
#737=PLANE('',#25300);
#738=PLANE('',#25328);
#739=PLANE('',#25331);
#740=PLANE('',#25335);
#741=PLANE('',#25337);
#742=PLANE('',#25345);
#743=PLANE('',#25372);
#744=PLANE('',#25375);
#745=PLANE('',#25379);
#746=PLANE('',#25383);
#747=PLANE('',#25396);
#748=PLANE('',#25409);
#749=PLANE('',#25412);
#750=PLANE('',#25415);
#751=PLANE('',#25416);
#752=PLANE('',#25419);
#753=PLANE('',#25422);
#754=PLANE('',#25423);
#755=PLANE('',#25428);
#756=PLANE('',#25432);
#757=PLANE('',#25437);
#758=PLANE('',#25438);
#759=PLANE('',#25439);
#760=PLANE('',#25440);
#761=PLANE('',#25441);
#762=PLANE('',#25442);
#763=PLANE('',#25443);
#1747=FACE_OUTER_BOUND('',#3078,.T.);
#1748=FACE_OUTER_BOUND('',#3079,.T.);
#1749=FACE_OUTER_BOUND('',#3081,.T.);
#1750=FACE_OUTER_BOUND('',#3082,.T.);
#1751=FACE_OUTER_BOUND('',#3083,.T.);
#1752=FACE_OUTER_BOUND('',#3085,.T.);
#1753=FACE_OUTER_BOUND('',#3086,.T.);
#1754=FACE_OUTER_BOUND('',#3087,.T.);
#1755=FACE_OUTER_BOUND('',#3088,.T.);
#1756=FACE_OUTER_BOUND('',#3090,.T.);
#1757=FACE_OUTER_BOUND('',#3091,.T.);
#1758=FACE_OUTER_BOUND('',#3093,.T.);
#1759=FACE_OUTER_BOUND('',#3094,.T.);
#1760=FACE_OUTER_BOUND('',#3095,.T.);
#1761=FACE_OUTER_BOUND('',#3096,.T.);
#1762=FACE_OUTER_BOUND('',#3103,.T.);
#1763=FACE_OUTER_BOUND('',#3104,.T.);
#1764=FACE_OUTER_BOUND('',#3105,.T.);
#1765=FACE_OUTER_BOUND('',#3106,.T.);
#1766=FACE_OUTER_BOUND('',#3107,.T.);
#1767=FACE_OUTER_BOUND('',#3108,.T.);
#1768=FACE_OUTER_BOUND('',#3109,.T.);
#1769=FACE_OUTER_BOUND('',#3110,.T.);
#1770=FACE_OUTER_BOUND('',#3111,.T.);
#1771=FACE_OUTER_BOUND('',#3112,.T.);
#1772=FACE_OUTER_BOUND('',#3113,.T.);
#1773=FACE_OUTER_BOUND('',#3114,.T.);
#1774=FACE_OUTER_BOUND('',#3115,.T.);
#1775=FACE_OUTER_BOUND('',#3116,.T.);
#1776=FACE_OUTER_BOUND('',#3117,.T.);
#1777=FACE_OUTER_BOUND('',#3118,.T.);
#1778=FACE_OUTER_BOUND('',#3119,.T.);
#1779=FACE_OUTER_BOUND('',#3120,.T.);
#1780=FACE_OUTER_BOUND('',#3121,.T.);
#1781=FACE_OUTER_BOUND('',#3131,.T.);
#1782=FACE_OUTER_BOUND('',#3132,.T.);
#1783=FACE_OUTER_BOUND('',#3133,.T.);
#1784=FACE_OUTER_BOUND('',#3134,.T.);
#1785=FACE_OUTER_BOUND('',#3135,.T.);
#1786=FACE_OUTER_BOUND('',#3136,.T.);
#1787=FACE_OUTER_BOUND('',#3137,.T.);
#1788=FACE_OUTER_BOUND('',#3138,.T.);
#1789=FACE_OUTER_BOUND('',#3139,.T.);
#1790=FACE_OUTER_BOUND('',#3140,.T.);
#1791=FACE_OUTER_BOUND('',#3141,.T.);
#1792=FACE_OUTER_BOUND('',#3142,.T.);
#1793=FACE_OUTER_BOUND('',#3143,.T.);
#1794=FACE_OUTER_BOUND('',#3144,.T.);
#1795=FACE_OUTER_BOUND('',#3145,.T.);
#1796=FACE_OUTER_BOUND('',#3146,.T.);
#1797=FACE_OUTER_BOUND('',#3147,.T.);
#1798=FACE_OUTER_BOUND('',#3148,.T.);
#1799=FACE_OUTER_BOUND('',#3149,.T.);
#1800=FACE_OUTER_BOUND('',#3150,.T.);
#1801=FACE_OUTER_BOUND('',#3151,.T.);
#1802=FACE_OUTER_BOUND('',#3152,.T.);
#1803=FACE_OUTER_BOUND('',#3153,.T.);
#1804=FACE_OUTER_BOUND('',#3154,.T.);
#1805=FACE_OUTER_BOUND('',#3155,.T.);
#1806=FACE_OUTER_BOUND('',#3156,.T.);
#1807=FACE_OUTER_BOUND('',#3157,.T.);
#1808=FACE_OUTER_BOUND('',#3158,.T.);
#1809=FACE_OUTER_BOUND('',#3159,.T.);
#1810=FACE_OUTER_BOUND('',#3160,.T.);
#1811=FACE_OUTER_BOUND('',#3161,.T.);
#1812=FACE_OUTER_BOUND('',#3162,.T.);
#1813=FACE_OUTER_BOUND('',#3163,.T.);
#1814=FACE_OUTER_BOUND('',#3164,.T.);
#1815=FACE_OUTER_BOUND('',#3165,.T.);
#1816=FACE_OUTER_BOUND('',#3166,.T.);
#1817=FACE_OUTER_BOUND('',#3167,.T.);
#1818=FACE_OUTER_BOUND('',#3168,.T.);
#1819=FACE_OUTER_BOUND('',#3169,.T.);
#1820=FACE_OUTER_BOUND('',#3170,.T.);
#1821=FACE_OUTER_BOUND('',#3171,.T.);
#1822=FACE_OUTER_BOUND('',#3172,.T.);
#1823=FACE_OUTER_BOUND('',#3173,.T.);
#1824=FACE_OUTER_BOUND('',#3174,.T.);
#1825=FACE_OUTER_BOUND('',#3175,.T.);
#1826=FACE_OUTER_BOUND('',#3176,.T.);
#1827=FACE_OUTER_BOUND('',#3177,.T.);
#1828=FACE_OUTER_BOUND('',#3178,.T.);
#1829=FACE_OUTER_BOUND('',#3179,.T.);
#1830=FACE_OUTER_BOUND('',#3180,.T.);
#1831=FACE_OUTER_BOUND('',#3181,.T.);
#1832=FACE_OUTER_BOUND('',#3182,.T.);
#1833=FACE_OUTER_BOUND('',#3183,.T.);
#1834=FACE_OUTER_BOUND('',#3184,.T.);
#1835=FACE_OUTER_BOUND('',#3185,.T.);
#1836=FACE_OUTER_BOUND('',#3186,.T.);
#1837=FACE_OUTER_BOUND('',#3187,.T.);
#1838=FACE_OUTER_BOUND('',#3188,.T.);
#1839=FACE_OUTER_BOUND('',#3189,.T.);
#1840=FACE_OUTER_BOUND('',#3190,.T.);
#1841=FACE_OUTER_BOUND('',#3191,.T.);
#1842=FACE_OUTER_BOUND('',#3192,.T.);
#1843=FACE_OUTER_BOUND('',#3193,.T.);
#1844=FACE_OUTER_BOUND('',#3194,.T.);
#1845=FACE_OUTER_BOUND('',#3195,.T.);
#1846=FACE_OUTER_BOUND('',#3196,.T.);
#1847=FACE_OUTER_BOUND('',#3197,.T.);
#1848=FACE_OUTER_BOUND('',#3198,.T.);
#1849=FACE_OUTER_BOUND('',#3199,.T.);
#1850=FACE_OUTER_BOUND('',#3200,.T.);
#1851=FACE_OUTER_BOUND('',#3201,.T.);
#1852=FACE_OUTER_BOUND('',#3202,.T.);
#1853=FACE_OUTER_BOUND('',#3203,.T.);
#1854=FACE_OUTER_BOUND('',#3204,.T.);
#1855=FACE_OUTER_BOUND('',#3205,.T.);
#1856=FACE_OUTER_BOUND('',#3206,.T.);
#1857=FACE_OUTER_BOUND('',#3207,.T.);
#1858=FACE_OUTER_BOUND('',#3208,.T.);
#1859=FACE_OUTER_BOUND('',#3209,.T.);
#1860=FACE_OUTER_BOUND('',#3210,.T.);
#1861=FACE_OUTER_BOUND('',#3211,.T.);
#1862=FACE_OUTER_BOUND('',#3212,.T.);
#1863=FACE_OUTER_BOUND('',#3213,.T.);
#1864=FACE_OUTER_BOUND('',#3214,.T.);
#1865=FACE_OUTER_BOUND('',#3215,.T.);
#1866=FACE_OUTER_BOUND('',#3216,.T.);
#1867=FACE_OUTER_BOUND('',#3217,.T.);
#1868=FACE_OUTER_BOUND('',#3218,.T.);
#1869=FACE_OUTER_BOUND('',#3219,.T.);
#1870=FACE_OUTER_BOUND('',#3220,.T.);
#1871=FACE_OUTER_BOUND('',#3221,.T.);
#1872=FACE_OUTER_BOUND('',#3222,.T.);
#1873=FACE_OUTER_BOUND('',#3223,.T.);
#1874=FACE_OUTER_BOUND('',#3224,.T.);
#1875=FACE_OUTER_BOUND('',#3225,.T.);
#1876=FACE_OUTER_BOUND('',#3226,.T.);
#1877=FACE_OUTER_BOUND('',#3227,.T.);
#1878=FACE_OUTER_BOUND('',#3229,.T.);
#1879=FACE_OUTER_BOUND('',#3230,.T.);
#1880=FACE_OUTER_BOUND('',#3231,.T.);
#1881=FACE_OUTER_BOUND('',#3232,.T.);
#1882=FACE_OUTER_BOUND('',#3233,.T.);
#1883=FACE_OUTER_BOUND('',#3234,.T.);
#1884=FACE_OUTER_BOUND('',#3235,.T.);
#1885=FACE_OUTER_BOUND('',#3236,.T.);
#1886=FACE_OUTER_BOUND('',#3237,.T.);
#1887=FACE_OUTER_BOUND('',#3238,.T.);
#1888=FACE_OUTER_BOUND('',#3239,.T.);
#1889=FACE_OUTER_BOUND('',#3240,.T.);
#1890=FACE_OUTER_BOUND('',#3241,.T.);
#1891=FACE_OUTER_BOUND('',#3242,.T.);
#1892=FACE_OUTER_BOUND('',#3243,.T.);
#1893=FACE_OUTER_BOUND('',#3244,.T.);
#1894=FACE_OUTER_BOUND('',#3245,.T.);
#1895=FACE_OUTER_BOUND('',#3246,.T.);
#1896=FACE_OUTER_BOUND('',#3247,.T.);
#1897=FACE_OUTER_BOUND('',#3248,.T.);
#1898=FACE_OUTER_BOUND('',#3249,.T.);
#1899=FACE_OUTER_BOUND('',#3250,.T.);
#1900=FACE_OUTER_BOUND('',#3251,.T.);
#1901=FACE_OUTER_BOUND('',#3252,.T.);
#1902=FACE_OUTER_BOUND('',#3253,.T.);
#1903=FACE_OUTER_BOUND('',#3255,.T.);
#1904=FACE_OUTER_BOUND('',#3256,.T.);
#1905=FACE_OUTER_BOUND('',#3257,.T.);
#1906=FACE_OUTER_BOUND('',#3258,.T.);
#1907=FACE_OUTER_BOUND('',#3259,.T.);
#1908=FACE_OUTER_BOUND('',#3261,.T.);
#1909=FACE_OUTER_BOUND('',#3262,.T.);
#1910=FACE_OUTER_BOUND('',#3264,.T.);
#1911=FACE_OUTER_BOUND('',#3265,.T.);
#1912=FACE_OUTER_BOUND('',#3266,.T.);
#1913=FACE_OUTER_BOUND('',#3269,.T.);
#1914=FACE_OUTER_BOUND('',#3270,.T.);
#1915=FACE_OUTER_BOUND('',#3271,.T.);
#1916=FACE_OUTER_BOUND('',#3272,.T.);
#1917=FACE_OUTER_BOUND('',#3273,.T.);
#1918=FACE_OUTER_BOUND('',#3274,.T.);
#1919=FACE_OUTER_BOUND('',#3275,.T.);
#1920=FACE_OUTER_BOUND('',#3276,.T.);
#1921=FACE_OUTER_BOUND('',#3277,.T.);
#1922=FACE_OUTER_BOUND('',#3278,.T.);
#3078=EDGE_LOOP('',(#16528,#16529,#16530,#16531));
#3079=EDGE_LOOP('',(#16532));
#3080=EDGE_LOOP('',(#16533));
#3081=EDGE_LOOP('',(#16534,#16535,#16536,#16537));
#3082=EDGE_LOOP('',(#16538,#16539,#16540,#16541));
#3083=EDGE_LOOP('',(#16542));
#3084=EDGE_LOOP('',(#16543));
#3085=EDGE_LOOP('',(#16544,#16545,#16546,#16547));
#3086=EDGE_LOOP('',(#16548,#16549,#16550,#16551,#16552));
#3087=EDGE_LOOP('',(#16553,#16554,#16555,#16556,#16557));
#3088=EDGE_LOOP('',(#16558));
#3089=EDGE_LOOP('',(#16559));
#3090=EDGE_LOOP('',(#16560,#16561,#16562,#16563));
#3091=EDGE_LOOP('',(#16564,#16565,#16566,#16567));
#3092=EDGE_LOOP('',(#16568));
#3093=EDGE_LOOP('',(#16569,#16570,#16571,#16572));
#3094=EDGE_LOOP('',(#16573,#16574,#16575,#16576));
#3095=EDGE_LOOP('',(#16577,#16578,#16579,#16580));
#3096=EDGE_LOOP('',(#16581,#16582,#16583,#16584,#16585,#16586,#16587,#16588,
#16589,#16590));
#3097=EDGE_LOOP('',(#16591));
#3098=EDGE_LOOP('',(#16592,#16593,#16594,#16595,#16596,#16597,#16598,#16599,
#16600,#16601,#16602,#16603,#16604,#16605,#16606,#16607,#16608,#16609,#16610,
#16611,#16612,#16613,#16614,#16615));
#3099=EDGE_LOOP('',(#16616,#16617,#16618,#16619,#16620));
#3100=EDGE_LOOP('',(#16621,#16622,#16623,#16624,#16625));
#3101=EDGE_LOOP('',(#16626,#16627,#16628,#16629,#16630));
#3102=EDGE_LOOP('',(#16631));
#3103=EDGE_LOOP('',(#16632,#16633,#16634,#16635,#16636,#16637));
#3104=EDGE_LOOP('',(#16638,#16639,#16640,#16641));
#3105=EDGE_LOOP('',(#16642,#16643,#16644,#16645));
#3106=EDGE_LOOP('',(#16646,#16647,#16648,#16649));
#3107=EDGE_LOOP('',(#16650,#16651,#16652,#16653));
#3108=EDGE_LOOP('',(#16654,#16655,#16656,#16657,#16658));
#3109=EDGE_LOOP('',(#16659,#16660,#16661,#16662));
#3110=EDGE_LOOP('',(#16663,#16664,#16665,#16666));
#3111=EDGE_LOOP('',(#16667,#16668,#16669,#16670));
#3112=EDGE_LOOP('',(#16671,#16672,#16673,#16674));
#3113=EDGE_LOOP('',(#16675,#16676,#16677,#16678));
#3114=EDGE_LOOP('',(#16679,#16680,#16681,#16682));
#3115=EDGE_LOOP('',(#16683,#16684,#16685,#16686,#16687,#16688,#16689,#16690,
#16691,#16692));
#3116=EDGE_LOOP('',(#16693,#16694,#16695,#16696));
#3117=EDGE_LOOP('',(#16697,#16698,#16699,#16700,#16701,#16702,#16703,#16704,
#16705,#16706));
#3118=EDGE_LOOP('',(#16707,#16708,#16709,#16710));
#3119=EDGE_LOOP('',(#16711,#16712,#16713,#16714));
#3120=EDGE_LOOP('',(#16715,#16716,#16717,#16718));
#3121=EDGE_LOOP('',(#16719,#16720,#16721,#16722,#16723,#16724,#16725,#16726));
#3122=EDGE_LOOP('',(#16727));
#3123=EDGE_LOOP('',(#16728));
#3124=EDGE_LOOP('',(#16729));
#3125=EDGE_LOOP('',(#16730,#16731,#16732,#16733));
#3126=EDGE_LOOP('',(#16734));
#3127=EDGE_LOOP('',(#16735));
#3128=EDGE_LOOP('',(#16736));
#3129=EDGE_LOOP('',(#16737));
#3130=EDGE_LOOP('',(#16738));
#3131=EDGE_LOOP('',(#16739,#16740,#16741,#16742));
#3132=EDGE_LOOP('',(#16743,#16744,#16745,#16746));
#3133=EDGE_LOOP('',(#16747,#16748,#16749,#16750));
#3134=EDGE_LOOP('',(#16751,#16752,#16753,#16754));
#3135=EDGE_LOOP('',(#16755,#16756,#16757,#16758));
#3136=EDGE_LOOP('',(#16759,#16760,#16761,#16762));
#3137=EDGE_LOOP('',(#16763,#16764,#16765,#16766));
#3138=EDGE_LOOP('',(#16767,#16768,#16769,#16770));
#3139=EDGE_LOOP('',(#16771,#16772,#16773,#16774));
#3140=EDGE_LOOP('',(#16775,#16776,#16777,#16778));
#3141=EDGE_LOOP('',(#16779,#16780,#16781,#16782,#16783,#16784));
#3142=EDGE_LOOP('',(#16785,#16786,#16787,#16788));
#3143=EDGE_LOOP('',(#16789,#16790,#16791,#16792));
#3144=EDGE_LOOP('',(#16793,#16794,#16795,#16796));
#3145=EDGE_LOOP('',(#16797,#16798,#16799,#16800));
#3146=EDGE_LOOP('',(#16801,#16802,#16803,#16804,#16805));
#3147=EDGE_LOOP('',(#16806,#16807,#16808,#16809));
#3148=EDGE_LOOP('',(#16810,#16811,#16812,#16813));
#3149=EDGE_LOOP('',(#16814,#16815,#16816,#16817));
#3150=EDGE_LOOP('',(#16818,#16819,#16820,#16821));
#3151=EDGE_LOOP('',(#16822,#16823,#16824,#16825));
#3152=EDGE_LOOP('',(#16826,#16827,#16828,#16829));
#3153=EDGE_LOOP('',(#16830,#16831,#16832,#16833));
#3154=EDGE_LOOP('',(#16834,#16835,#16836,#16837));
#3155=EDGE_LOOP('',(#16838,#16839,#16840,#16841,#16842,#16843));
#3156=EDGE_LOOP('',(#16844,#16845,#16846,#16847));
#3157=EDGE_LOOP('',(#16848,#16849,#16850,#16851));
#3158=EDGE_LOOP('',(#16852,#16853,#16854,#16855));
#3159=EDGE_LOOP('',(#16856,#16857,#16858,#16859));
#3160=EDGE_LOOP('',(#16860,#16861,#16862,#16863));
#3161=EDGE_LOOP('',(#16864,#16865,#16866,#16867));
#3162=EDGE_LOOP('',(#16868,#16869,#16870,#16871));
#3163=EDGE_LOOP('',(#16872,#16873,#16874,#16875));
#3164=EDGE_LOOP('',(#16876,#16877,#16878,#16879));
#3165=EDGE_LOOP('',(#16880,#16881,#16882,#16883));
#3166=EDGE_LOOP('',(#16884,#16885,#16886,#16887));
#3167=EDGE_LOOP('',(#16888,#16889,#16890,#16891));
#3168=EDGE_LOOP('',(#16892,#16893,#16894,#16895));
#3169=EDGE_LOOP('',(#16896,#16897,#16898,#16899));
#3170=EDGE_LOOP('',(#16900,#16901,#16902,#16903));
#3171=EDGE_LOOP('',(#16904,#16905,#16906,#16907));
#3172=EDGE_LOOP('',(#16908,#16909,#16910,#16911));
#3173=EDGE_LOOP('',(#16912,#16913,#16914,#16915));
#3174=EDGE_LOOP('',(#16916,#16917,#16918,#16919));
#3175=EDGE_LOOP('',(#16920,#16921,#16922,#16923));
#3176=EDGE_LOOP('',(#16924,#16925,#16926,#16927));
#3177=EDGE_LOOP('',(#16928,#16929,#16930,#16931));
#3178=EDGE_LOOP('',(#16932,#16933,#16934,#16935));
#3179=EDGE_LOOP('',(#16936,#16937,#16938,#16939));
#3180=EDGE_LOOP('',(#16940,#16941,#16942,#16943));
#3181=EDGE_LOOP('',(#16944,#16945,#16946,#16947));
#3182=EDGE_LOOP('',(#16948,#16949,#16950,#16951));
#3183=EDGE_LOOP('',(#16952,#16953,#16954,#16955));
#3184=EDGE_LOOP('',(#16956,#16957,#16958,#16959));
#3185=EDGE_LOOP('',(#16960,#16961,#16962,#16963));
#3186=EDGE_LOOP('',(#16964,#16965,#16966,#16967));
#3187=EDGE_LOOP('',(#16968,#16969,#16970,#16971));
#3188=EDGE_LOOP('',(#16972,#16973,#16974,#16975));
#3189=EDGE_LOOP('',(#16976,#16977,#16978,#16979));
#3190=EDGE_LOOP('',(#16980,#16981,#16982,#16983));
#3191=EDGE_LOOP('',(#16984,#16985,#16986,#16987));
#3192=EDGE_LOOP('',(#16988,#16989,#16990,#16991));
#3193=EDGE_LOOP('',(#16992,#16993,#16994,#16995));
#3194=EDGE_LOOP('',(#16996,#16997,#16998,#16999));
#3195=EDGE_LOOP('',(#17000,#17001,#17002,#17003));
#3196=EDGE_LOOP('',(#17004,#17005,#17006,#17007));
#3197=EDGE_LOOP('',(#17008,#17009,#17010,#17011));
#3198=EDGE_LOOP('',(#17012,#17013,#17014,#17015));
#3199=EDGE_LOOP('',(#17016,#17017,#17018,#17019));
#3200=EDGE_LOOP('',(#17020,#17021,#17022,#17023));
#3201=EDGE_LOOP('',(#17024,#17025,#17026,#17027));
#3202=EDGE_LOOP('',(#17028,#17029,#17030,#17031));
#3203=EDGE_LOOP('',(#17032,#17033,#17034,#17035));
#3204=EDGE_LOOP('',(#17036,#17037,#17038,#17039));
#3205=EDGE_LOOP('',(#17040,#17041,#17042,#17043));
#3206=EDGE_LOOP('',(#17044,#17045,#17046,#17047));
#3207=EDGE_LOOP('',(#17048,#17049,#17050,#17051));
#3208=EDGE_LOOP('',(#17052,#17053,#17054,#17055));
#3209=EDGE_LOOP('',(#17056,#17057,#17058,#17059));
#3210=EDGE_LOOP('',(#17060,#17061,#17062,#17063));
#3211=EDGE_LOOP('',(#17064,#17065,#17066,#17067));
#3212=EDGE_LOOP('',(#17068,#17069,#17070,#17071,#17072));
#3213=EDGE_LOOP('',(#17073,#17074,#17075,#17076));
#3214=EDGE_LOOP('',(#17077,#17078,#17079,#17080));
#3215=EDGE_LOOP('',(#17081,#17082,#17083,#17084));
#3216=EDGE_LOOP('',(#17085,#17086,#17087,#17088));
#3217=EDGE_LOOP('',(#17089,#17090,#17091,#17092));
#3218=EDGE_LOOP('',(#17093,#17094,#17095,#17096));
#3219=EDGE_LOOP('',(#17097,#17098,#17099,#17100));
#3220=EDGE_LOOP('',(#17101,#17102,#17103,#17104));
#3221=EDGE_LOOP('',(#17105,#17106,#17107,#17108));
#3222=EDGE_LOOP('',(#17109,#17110,#17111,#17112));
#3223=EDGE_LOOP('',(#17113,#17114,#17115,#17116));
#3224=EDGE_LOOP('',(#17117,#17118,#17119,#17120));
#3225=EDGE_LOOP('',(#17121,#17122,#17123,#17124));
#3226=EDGE_LOOP('',(#17125,#17126,#17127,#17128,#17129,#17130,#17131,#17132,
#17133,#17134,#17135,#17136,#17137,#17138,#17139,#17140));
#3227=EDGE_LOOP('',(#17141));
#3228=EDGE_LOOP('',(#17142));
#3229=EDGE_LOOP('',(#17143,#17144,#17145,#17146,#17147));
#3230=EDGE_LOOP('',(#17148,#17149,#17150,#17151));
#3231=EDGE_LOOP('',(#17152,#17153,#17154,#17155,#17156,#17157));
#3232=EDGE_LOOP('',(#17158,#17159,#17160,#17161,#17162,#17163));
#3233=EDGE_LOOP('',(#17164,#17165,#17166));
#3234=EDGE_LOOP('',(#17167,#17168,#17169,#17170,#17171,#17172,#17173));
#3235=EDGE_LOOP('',(#17174,#17175,#17176,#17177,#17178,#17179));
#3236=EDGE_LOOP('',(#17180,#17181));
#3237=EDGE_LOOP('',(#17182,#17183,#17184,#17185));
#3238=EDGE_LOOP('',(#17186,#17187,#17188,#17189));
#3239=EDGE_LOOP('',(#17190,#17191,#17192,#17193));
#3240=EDGE_LOOP('',(#17194,#17195,#17196,#17197));
#3241=EDGE_LOOP('',(#17198,#17199,#17200,#17201));
#3242=EDGE_LOOP('',(#17202,#17203,#17204,#17205));
#3243=EDGE_LOOP('',(#17206,#17207,#17208,#17209));
#3244=EDGE_LOOP('',(#17210,#17211,#17212,#17213));
#3245=EDGE_LOOP('',(#17214,#17215,#17216,#17217));
#3246=EDGE_LOOP('',(#17218,#17219,#17220,#17221));
#3247=EDGE_LOOP('',(#17222,#17223,#17224,#17225));
#3248=EDGE_LOOP('',(#17226,#17227,#17228,#17229));
#3249=EDGE_LOOP('',(#17230,#17231,#17232,#17233));
#3250=EDGE_LOOP('',(#17234,#17235,#17236,#17237));
#3251=EDGE_LOOP('',(#17238,#17239,#17240,#17241));
#3252=EDGE_LOOP('',(#17242,#17243,#17244,#17245));
#3253=EDGE_LOOP('',(#17246,#17247,#17248,#17249));
#3254=EDGE_LOOP('',(#17250,#17251,#17252,#17253));
#3255=EDGE_LOOP('',(#17254,#17255,#17256,#17257));
#3256=EDGE_LOOP('',(#17258));
#3257=EDGE_LOOP('',(#17259,#17260,#17261,#17262));
#3258=EDGE_LOOP('',(#17263));
#3259=EDGE_LOOP('',(#17264));
#3260=EDGE_LOOP('',(#17265));
#3261=EDGE_LOOP('',(#17266,#17267,#17268,#17269));
#3262=EDGE_LOOP('',(#17270));
#3263=EDGE_LOOP('',(#17271));
#3264=EDGE_LOOP('',(#17272,#17273,#17274,#17275));
#3265=EDGE_LOOP('',(#17276,#17277,#17278,#17279));
#3266=EDGE_LOOP('',(#17280,#17281,#17282,#17283,#17284,#17285,#17286,#17287,
#17288,#17289,#17290,#17291,#17292,#17293,#17294,#17295,#17296,#17297,#17298,
#17299,#17300,#17301,#17302,#17303,#17304,#17305));
#3267=EDGE_LOOP('',(#17306));
#3268=EDGE_LOOP('',(#17307));
#3269=EDGE_LOOP('',(#17308,#17309,#17310,#17311));
#3270=EDGE_LOOP('',(#17312,#17313,#17314,#17315));
#3271=EDGE_LOOP('',(#17316,#17317));
#3272=EDGE_LOOP('',(#17318,#17319,#17320,#17321,#17322,#17323,#17324,#17325,
#17326,#17327));
#3273=EDGE_LOOP('',(#17328,#17329,#17330,#17331));
#3274=EDGE_LOOP('',(#17332,#17333,#17334,#17335));
#3275=EDGE_LOOP('',(#17336,#17337,#17338,#17339,#17340));
#3276=EDGE_LOOP('',(#17341,#17342,#17343,#17344,#17345));
#3277=EDGE_LOOP('',(#17346,#17347,#17348,#17349));
#3278=EDGE_LOOP('',(#17350,#17351,#17352,#17353));
#4534=LINE('',#33462,#7403);
#4535=LINE('',#33469,#7404);
#4536=LINE('',#33475,#7405);
#4537=LINE('',#33482,#7406);
#4538=LINE('',#33488,#7407);
#4539=LINE('',#33494,#7408);
#4540=LINE('',#33502,#7409);
#4541=LINE('',#33506,#7410);
#4542=LINE('',#33510,#7411);
#4543=LINE('',#33654,#7412);
#4544=LINE('',#33687,#7413);
#4545=LINE('',#33697,#7414);
#4546=LINE('',#33698,#7415);
#4547=LINE('',#33699,#7416);
#4548=LINE('',#33703,#7417);
#4549=LINE('',#33707,#7418);
#4550=LINE('',#33711,#7419);
#4551=LINE('',#33715,#7420);
#4552=LINE('',#33719,#7421);
#4553=LINE('',#33724,#7422);
#4554=LINE('',#33726,#7423);
#4555=LINE('',#33728,#7424);
#4556=LINE('',#33732,#7425);
#4557=LINE('',#33734,#7426);
#4558=LINE('',#33736,#7427);
#4559=LINE('',#33742,#7428);
#4560=LINE('',#33746,#7429);
#4561=LINE('',#33750,#7430);
#4562=LINE('',#33756,#7431);
#4563=LINE('',#33758,#7432);
#4564=LINE('',#33760,#7433);
#4565=LINE('',#33762,#7434);
#4566=LINE('',#33764,#7435);
#4567=LINE('',#33767,#7436);
#4568=LINE('',#33772,#7437);
#4569=LINE('',#33777,#7438);
#4570=LINE('',#33792,#7439);
#4571=LINE('',#33797,#7440);
#4572=LINE('',#33802,#7441);
#4573=LINE('',#33868,#7442);
#4574=LINE('',#33869,#7443);
#4575=LINE('',#33983,#7444);
#4576=LINE('',#33993,#7445);
#4577=LINE('',#33994,#7446);
#4578=LINE('',#33997,#7447);
#4579=LINE('',#34014,#7448);
#4580=LINE('',#34015,#7449);
#4581=LINE('',#34018,#7450);
#4582=LINE('',#34023,#7451);
#4583=LINE('',#34026,#7452);
#4584=LINE('',#34031,#7453);
#4585=LINE('',#34042,#7454);
#4586=LINE('',#34050,#7455);
#4587=LINE('',#34055,#7456);
#4588=LINE('',#34069,#7457);
#4589=LINE('',#34090,#7458);
#4590=LINE('',#34098,#7459);
#4591=LINE('',#34103,#7460);
#4592=LINE('',#34126,#7461);
#4593=LINE('',#34143,#7462);
#4594=LINE('',#34159,#7463);
#4595=LINE('',#34163,#7464);
#4596=LINE('',#34169,#7465);
#4597=LINE('',#34173,#7466);
#4598=LINE('',#34177,#7467);
#4599=LINE('',#34180,#7468);
#4600=LINE('',#34189,#7469);
#4601=LINE('',#34193,#7470);
#4602=LINE('',#34204,#7471);
#4603=LINE('',#34206,#7472);
#4604=LINE('',#34208,#7473);
#4605=LINE('',#34211,#7474);
#4606=LINE('',#34216,#7475);
#4607=LINE('',#34219,#7476);
#4608=LINE('',#34224,#7477);
#4609=LINE('',#34397,#7478);
#4610=LINE('',#34407,#7479);
#4611=LINE('',#34408,#7480);
#4612=LINE('',#34409,#7481);
#4613=LINE('',#34412,#7482);
#4614=LINE('',#34477,#7483);
#4615=LINE('',#34478,#7484);
#4616=LINE('',#34588,#7485);
#4617=LINE('',#34597,#7486);
#4618=LINE('',#34598,#7487);
#4619=LINE('',#34601,#7488);
#4620=LINE('',#34618,#7489);
#4621=LINE('',#34619,#7490);
#4622=LINE('',#34621,#7491);
#4623=LINE('',#34623,#7492);
#4624=LINE('',#34627,#7493);
#4625=LINE('',#34629,#7494);
#4626=LINE('',#34631,#7495);
#4627=LINE('',#34632,#7496);
#4628=LINE('',#34635,#7497);
#4629=LINE('',#34640,#7498);
#4630=LINE('',#34641,#7499);
#4631=LINE('',#34645,#7500);
#4632=LINE('',#34651,#7501);
#4633=LINE('',#34652,#7502);
#4634=LINE('',#34653,#7503);
#4635=LINE('',#34655,#7504);
#4636=LINE('',#34689,#7505);
#4637=LINE('',#34692,#7506);
#4638=LINE('',#34749,#7507);
#4639=LINE('',#34751,#7508);
#4640=LINE('',#34754,#7509);
#4641=LINE('',#34757,#7510);
#4642=LINE('',#34760,#7511);
#4643=LINE('',#34761,#7512);
#4644=LINE('',#34764,#7513);
#4645=LINE('',#34822,#7514);
#4646=LINE('',#34824,#7515);
#4647=LINE('',#34827,#7516);
#4648=LINE('',#34830,#7517);
#4649=LINE('',#34833,#7518);
#4650=LINE('',#34834,#7519);
#4651=LINE('',#34837,#7520);
#4652=LINE('',#34888,#7521);
#4653=LINE('',#34923,#7522);
#4654=LINE('',#34926,#7523);
#4655=LINE('',#34930,#7524);
#4656=LINE('',#34987,#7525);
#4657=LINE('',#34993,#7526);
#4658=LINE('',#34996,#7527);
#4659=LINE('',#34997,#7528);
#4660=LINE('',#35000,#7529);
#4661=LINE('',#35004,#7530);
#4662=LINE('',#35005,#7531);
#4663=LINE('',#35008,#7532);
#4664=LINE('',#35012,#7533);
#4665=LINE('',#35013,#7534);
#4666=LINE('',#35016,#7535);
#4667=LINE('',#35020,#7536);
#4668=LINE('',#35026,#7537);
#4669=LINE('',#35035,#7538);
#4670=LINE('',#35043,#7539);
#4671=LINE('',#35049,#7540);
#4672=LINE('',#35055,#7541);
#4673=LINE('',#35058,#7542);
#4674=LINE('',#35061,#7543);
#4675=LINE('',#35064,#7544);
#4676=LINE('',#35065,#7545);
#4677=LINE('',#35068,#7546);
#4678=LINE('',#35072,#7547);
#4679=LINE('',#35073,#7548);
#4680=LINE('',#35076,#7549);
#4681=LINE('',#35079,#7550);
#4682=LINE('',#35081,#7551);
#4683=LINE('',#35083,#7552);
#4684=LINE('',#35085,#7553);
#4685=LINE('',#35119,#7554);
#4686=LINE('',#35125,#7555);
#4687=LINE('',#35128,#7556);
#4688=LINE('',#35129,#7557);
#4689=LINE('',#35146,#7558);
#4690=LINE('',#35152,#7559);
#4691=LINE('',#35184,#7560);
#4692=LINE('',#35195,#7561);
#4693=LINE('',#35197,#7562);
#4694=LINE('',#35210,#7563);
#4695=LINE('',#35219,#7564);
#4696=LINE('',#35224,#7565);
#4697=LINE('',#35227,#7566);
#4698=LINE('',#35230,#7567);
#4699=LINE('',#35231,#7568);
#4700=LINE('',#35236,#7569);
#4701=LINE('',#35245,#7570);
#4702=LINE('',#35250,#7571);
#4703=LINE('',#35253,#7572);
#4704=LINE('',#35256,#7573);
#4705=LINE('',#35257,#7574);
#4706=LINE('',#35260,#7575);
#4707=LINE('',#35263,#7576);
#4708=LINE('',#35266,#7577);
#4709=LINE('',#35269,#7578);
#4710=LINE('',#35273,#7579);
#4711=LINE('',#35278,#7580);
#4712=LINE('',#35288,#7581);
#4713=LINE('',#35294,#7582);
#4714=LINE('',#35296,#7583);
#4715=LINE('',#35301,#7584);
#4716=LINE('',#35305,#7585);
#4717=LINE('',#35307,#7586);
#4718=LINE('',#35309,#7587);
#4719=LINE('',#35311,#7588);
#4720=LINE('',#35313,#7589);
#4721=LINE('',#35317,#7590);
#7403=VECTOR('',#26941,8.75);
#7404=VECTOR('',#26950,9.);
#7405=VECTOR('',#26957,8.75);
#7406=VECTOR('',#26966,9.);
#7407=VECTOR('',#26973,10.25);
#7408=VECTOR('',#26980,10.);
#7409=VECTOR('',#26991,10.25);
#7410=VECTOR('',#26994,10.);
#7411=VECTOR('',#26997,10.);
#7412=VECTOR('',#27000,10.);
#7413=VECTOR('',#27001,10.);
#7414=VECTOR('',#27004,10.);
#7415=VECTOR('',#27005,10.);
#7416=VECTOR('',#27006,10.);
#7417=VECTOR('',#27009,10.);
#7418=VECTOR('',#27012,10.);
#7419=VECTOR('',#27015,10.);
#7420=VECTOR('',#27018,10.);
#7421=VECTOR('',#27021,10.);
#7422=VECTOR('',#27026,10.);
#7423=VECTOR('',#27027,10.);
#7424=VECTOR('',#27028,10.);
#7425=VECTOR('',#27031,10.);
#7426=VECTOR('',#27032,10.);
#7427=VECTOR('',#27033,10.);
#7428=VECTOR('',#27038,10.);
#7429=VECTOR('',#27041,10.);
#7430=VECTOR('',#27044,10.);
#7431=VECTOR('',#27049,10.);
#7432=VECTOR('',#27050,10.);
#7433=VECTOR('',#27051,10.);
#7434=VECTOR('',#27052,10.);
#7435=VECTOR('',#27053,10.);
#7436=VECTOR('',#27056,10.);
#7437=VECTOR('',#27059,10.);
#7438=VECTOR('',#27064,10.);
#7439=VECTOR('',#27077,10.);
#7440=VECTOR('',#27082,10.);
#7441=VECTOR('',#27087,10.);
#7442=VECTOR('',#27090,10.);
#7443=VECTOR('',#27091,10.);
#7444=VECTOR('',#27092,10.);
#7445=VECTOR('',#27095,10.);
#7446=VECTOR('',#27096,10.);
#7447=VECTOR('',#27099,10.);
#7448=VECTOR('',#27102,10.);
#7449=VECTOR('',#27103,10.);
#7450=VECTOR('',#27106,5.3);
#7451=VECTOR('',#27113,5.05);
#7452=VECTOR('',#27116,5.3);
#7453=VECTOR('',#27123,5.05);
#7454=VECTOR('',#27126,10.);
#7455=VECTOR('',#27127,10.);
#7456=VECTOR('',#27132,5.05);
#7457=VECTOR('',#27137,10.);
#7458=VECTOR('',#27142,10.);
#7459=VECTOR('',#27143,10.);
#7460=VECTOR('',#27148,5.05);
#7461=VECTOR('',#27153,10.);
#7462=VECTOR('',#27158,10.);
#7463=VECTOR('',#27161,10.);
#7464=VECTOR('',#27166,5.3);
#7465=VECTOR('',#27171,10.);
#7466=VECTOR('',#27174,10.);
#7467=VECTOR('',#27177,10.);
#7468=VECTOR('',#27180,10.);
#7469=VECTOR('',#27187,10.);
#7470=VECTOR('',#27190,10.);
#7471=VECTOR('',#27203,5.3);
#7472=VECTOR('',#27206,5.3);
#7473=VECTOR('',#27209,5.3);
#7474=VECTOR('',#27212,5.75);
#7475=VECTOR('',#27219,5.5);
#7476=VECTOR('',#27222,5.75);
#7477=VECTOR('',#27229,5.5);
#7478=VECTOR('',#27230,10.);
#7479=VECTOR('',#27233,10.);
#7480=VECTOR('',#27234,10.);
#7481=VECTOR('',#27235,10.);
#7482=VECTOR('',#27238,10.);
#7483=VECTOR('',#27241,10.);
#7484=VECTOR('',#27242,10.);
#7485=VECTOR('',#27243,10.);
#7486=VECTOR('',#27246,10.);
#7487=VECTOR('',#27247,10.);
#7488=VECTOR('',#27250,10.);
#7489=VECTOR('',#27253,10.);
#7490=VECTOR('',#27254,10.);
#7491=VECTOR('',#27257,5.75);
#7492=VECTOR('',#27260,5.75);
#7493=VECTOR('',#27263,10.);
#7494=VECTOR('',#27264,10.);
#7495=VECTOR('',#27265,10.);
#7496=VECTOR('',#27266,10.);
#7497=VECTOR('',#27269,10.);
#7498=VECTOR('',#27276,10.);
#7499=VECTOR('',#27277,10.);
#7500=VECTOR('',#27280,10.);
#7501=VECTOR('',#27287,10.);
#7502=VECTOR('',#27288,10.);
#7503=VECTOR('',#27289,10.);
#7504=VECTOR('',#27292,10.);
#7505=VECTOR('',#27301,10.);
#7506=VECTOR('',#27304,10.);
#7507=VECTOR('',#27323,10.);
#7508=VECTOR('',#27326,10.);
#7509=VECTOR('',#27329,10.);
#7510=VECTOR('',#27332,10.);
#7511=VECTOR('',#27335,10.);
#7512=VECTOR('',#27336,10.);
#7513=VECTOR('',#27339,10.);
#7514=VECTOR('',#27360,10.);
#7515=VECTOR('',#27363,10.);
#7516=VECTOR('',#27366,10.);
#7517=VECTOR('',#27369,10.);
#7518=VECTOR('',#27372,10.);
#7519=VECTOR('',#27373,10.);
#7520=VECTOR('',#27376,10.);
#7521=VECTOR('',#27389,10.);
#7522=VECTOR('',#27396,10.);
#7523=VECTOR('',#27399,10.);
#7524=VECTOR('',#27402,10.);
#7525=VECTOR('',#27423,10.);
#7526=VECTOR('',#27432,10.);
#7527=VECTOR('',#27435,10.);
#7528=VECTOR('',#27436,10.);
#7529=VECTOR('',#27439,10.);
#7530=VECTOR('',#27444,10.);
#7531=VECTOR('',#27445,10.);
#7532=VECTOR('',#27448,10.);
#7533=VECTOR('',#27453,10.);
#7534=VECTOR('',#27454,10.);
#7535=VECTOR('',#27457,10.);
#7536=VECTOR('',#27462,10.);
#7537=VECTOR('',#27469,10.);
#7538=VECTOR('',#27482,10.);
#7539=VECTOR('',#27493,10.);
#7540=VECTOR('',#27502,10.);
#7541=VECTOR('',#27511,10.);
#7542=VECTOR('',#27514,10.);
#7543=VECTOR('',#27517,10.);
#7544=VECTOR('',#27520,10.);
#7545=VECTOR('',#27521,10.);
#7546=VECTOR('',#27524,10.);
#7547=VECTOR('',#27529,10.);
#7548=VECTOR('',#27530,10.);
#7549=VECTOR('',#27533,10.);
#7550=VECTOR('',#27538,10.);
#7551=VECTOR('',#27541,10.);
#7552=VECTOR('',#27544,10.);
#7553=VECTOR('',#27547,10.);
#7554=VECTOR('',#27554,10.);
#7555=VECTOR('',#27563,10.);
#7556=VECTOR('',#27566,10.);
#7557=VECTOR('',#27567,10.);
#7558=VECTOR('',#27598,10.);
#7559=VECTOR('',#27607,10.);
#7560=VECTOR('',#27622,41.28);
#7561=VECTOR('',#27629,10.);
#7562=VECTOR('',#27632,10.);
#7563=VECTOR('',#27653,10.);
#7564=VECTOR('',#27666,10.);
#7565=VECTOR('',#27673,10.);
#7566=VECTOR('',#27676,10.);
#7567=VECTOR('',#27679,10.);
#7568=VECTOR('',#27680,10.);
#7569=VECTOR('',#27685,10.);
#7570=VECTOR('',#27698,10.);
#7571=VECTOR('',#27705,10.);
#7572=VECTOR('',#27708,10.);
#7573=VECTOR('',#27711,10.);
#7574=VECTOR('',#27712,10.);
#7575=VECTOR('',#27715,10.);
#7576=VECTOR('',#27720,10.);
#7577=VECTOR('',#27723,10.);
#7578=VECTOR('',#27728,10.);
#7579=VECTOR('',#27733,4.01);
#7580=VECTOR('',#27740,4.01);
#7581=VECTOR('',#27753,14.7);
#7582=VECTOR('',#27762,14.3);
#7583=VECTOR('',#27765,14.3);
#7584=VECTOR('',#27772,10.);
#7585=VECTOR('',#27777,10.);
#7586=VECTOR('',#27780,10.);
#7587=VECTOR('',#27783,10.);
#7588=VECTOR('',#27786,10.);
#7589=VECTOR('',#27789,10.);
#7590=VECTOR('',#27796,10.);
#10272=CIRCLE('',#25109,8.5);
#10273=CIRCLE('',#25110,9.);
#10274=CIRCLE('',#25112,5.55);
#10275=CIRCLE('',#25114,9.);
#10276=CIRCLE('',#25116,8.5);
#10277=CIRCLE('',#25117,9.);
#10278=CIRCLE('',#25119,5.55);
#10279=CIRCLE('',#25121,9.);
#10280=CIRCLE('',#25123,10.5);
#10281=CIRCLE('',#25124,10.);
#10282=CIRCLE('',#25125,10.);
#10283=CIRCLE('',#25127,10.);
#10284=CIRCLE('',#25129,14.3);
#10285=CIRCLE('',#25131,10.5);
#10286=CIRCLE('',#25133,20.95);
#10287=CIRCLE('',#25134,20.95);
#10288=CIRCLE('',#25137,26.5);
#10289=CIRCLE('',#25138,26.5);
#10290=CIRCLE('',#25139,26.5);
#10291=CIRCLE('',#25140,26.5);
#10292=CIRCLE('',#25141,45.5);
#10293=CIRCLE('',#25142,6.);
#10294=CIRCLE('',#25143,45.5);
#10295=CIRCLE('',#25144,45.5);
#10296=CIRCLE('',#25145,9.5);
#10297=CIRCLE('',#25146,23.5);
#10298=CIRCLE('',#25147,23.5);
#10299=CIRCLE('',#25148,9.5);
#10300=CIRCLE('',#25149,45.5);
#10301=CIRCLE('',#25150,45.5);
#10302=CIRCLE('',#25151,23.5);
#10303=CIRCLE('',#25152,9.5);
#10304=CIRCLE('',#25153,45.5);
#10305=CIRCLE('',#25154,6.55);
#10306=CIRCLE('',#25155,41.28);
#10307=CIRCLE('',#25156,41.28);
#10308=CIRCLE('',#25157,6.55);
#10309=CIRCLE('',#25158,41.28);
#10310=CIRCLE('',#25159,23.5);
#10311=CIRCLE('',#25160,45.5);
#10312=CIRCLE('',#25161,9.5);
#10313=CIRCLE('',#25162,6.);
#10314=CIRCLE('',#25169,5.05);
#10315=CIRCLE('',#25171,5.05);
#10316=CIRCLE('',#25173,5.05);
#10317=CIRCLE('',#25175,5.05);
#10318=CIRCLE('',#25178,5.05);
#10319=CIRCLE('',#25179,5.05);
#10320=CIRCLE('',#25180,5.05);
#10321=CIRCLE('',#25181,5.05);
#10322=CIRCLE('',#25184,5.05);
#10323=CIRCLE('',#25185,5.05);
#10324=CIRCLE('',#25186,5.05);
#10325=CIRCLE('',#25187,5.05);
#10326=CIRCLE('',#25191,5.55);
#10327=CIRCLE('',#25193,26.5);
#10328=CIRCLE('',#25194,26.5);
#10329=CIRCLE('',#25195,26.5);
#10330=CIRCLE('',#25196,26.5);
#10331=CIRCLE('',#25197,5.55);
#10332=CIRCLE('',#25198,5.55);
#10333=CIRCLE('',#25199,6.);
#10334=CIRCLE('',#25200,26.05);
#10335=CIRCLE('',#25201,26.05);
#10336=CIRCLE('',#25202,4.01);
#10337=CIRCLE('',#25203,4.01);
#10338=CIRCLE('',#25204,6.);
#10339=CIRCLE('',#25205,5.55);
#10340=CIRCLE('',#25210,5.5);
#10341=CIRCLE('',#25212,5.5);
#10342=CIRCLE('',#25214,5.5);
#10343=CIRCLE('',#25216,5.5);
#10344=CIRCLE('',#25227,1.5);
#10345=CIRCLE('',#25228,0.999999999999995);
#10346=CIRCLE('',#25231,1.5);
#10347=CIRCLE('',#25232,0.999999999999996);
#10348=CIRCLE('',#25236,47.);
#10349=CIRCLE('',#25237,45.5);
#10350=CIRCLE('',#25239,47.);
#10351=CIRCLE('',#25241,11.);
#10352=CIRCLE('',#25243,47.);
#10353=CIRCLE('',#25245,1.5);
#10354=CIRCLE('',#25246,22.);
#10355=CIRCLE('',#25247,1.5);
#10356=CIRCLE('',#25251,47.);
#10357=CIRCLE('',#25254,22.);
#10358=CIRCLE('',#25256,47.);
#10359=CIRCLE('',#25258,11.);
#10360=CIRCLE('',#25260,1.5);
#10361=CIRCLE('',#25261,22.);
#10362=CIRCLE('',#25262,1.5);
#10363=CIRCLE('',#25266,11.);
#10364=CIRCLE('',#25269,22.);
#10365=CIRCLE('',#25272,47.);
#10366=CIRCLE('',#25274,47.);
#10367=CIRCLE('',#25276,11.);
#10368=CIRCLE('',#25278,11.);
#10369=CIRCLE('',#25280,1.5);
#10370=CIRCLE('',#25282,11.);
#10371=CIRCLE('',#25284,47.);
#10372=CIRCLE('',#25286,1.49999999999999);
#10373=CIRCLE('',#25287,22.);
#10374=CIRCLE('',#25289,1.5);
#10375=CIRCLE('',#25291,1.5);
#10376=CIRCLE('',#25292,22.);
#10377=CIRCLE('',#25296,22.);
#10378=CIRCLE('',#25299,22.);
#10379=CIRCLE('',#25302,11.);
#10380=CIRCLE('',#25304,47.);
#10381=CIRCLE('',#25306,1.5);
#10382=CIRCLE('',#25307,1.5);
#10383=CIRCLE('',#25309,1.49999999999999);
#10384=CIRCLE('',#25310,28.);
#10385=CIRCLE('',#25312,1.5);
#10386=CIRCLE('',#25314,1.5);
#10387=CIRCLE('',#25315,28.);
#10388=CIRCLE('',#25317,1.5);
#10389=CIRCLE('',#25319,1.5);
#10390=CIRCLE('',#25320,28.);
#10391=CIRCLE('',#25323,1.5);
#10392=CIRCLE('',#25324,28.);
#10393=CIRCLE('',#25327,28.);
#10394=CIRCLE('',#25330,28.);
#10395=CIRCLE('',#25333,28.);
#10396=CIRCLE('',#25339,47.);
#10397=CIRCLE('',#25342,47.);
#10398=CIRCLE('',#25344,47.);
#10399=CIRCLE('',#25347,47.);
#10400=CIRCLE('',#25349,1.5);
#10401=CIRCLE('',#25350,1.49999999999999);
#10402=CIRCLE('',#25352,1.5);
#10403=CIRCLE('',#25354,1.49999999999999);
#10404=CIRCLE('',#25356,1.5);
#10405=CIRCLE('',#25358,1.49999999999999);
#10406=CIRCLE('',#25360,1.5);
#10407=CIRCLE('',#25362,1.5);
#10408=CIRCLE('',#25363,28.);
#10409=CIRCLE('',#25366,41.28);
#10410=CIRCLE('',#25367,1.5);
#10411=CIRCLE('',#25368,39.78);
#10412=CIRCLE('',#25370,41.28);
#10413=CIRCLE('',#25371,41.28);
#10414=CIRCLE('',#25373,14.3);
#10415=CIRCLE('',#25378,39.78);
#10416=CIRCLE('',#25382,39.78);
#10417=CIRCLE('',#25385,1.5);
#10418=CIRCLE('',#25386,1.5);
#10419=CIRCLE('',#25388,1.5);
#10420=CIRCLE('',#25389,24.55);
#10421=CIRCLE('',#25391,1.5);
#10422=CIRCLE('',#25393,24.55);
#10423=CIRCLE('',#25395,24.55);
#10424=CIRCLE('',#25398,1.5);
#10425=CIRCLE('',#25399,1.5);
#10426=CIRCLE('',#25401,1.5);
#10427=CIRCLE('',#25402,22.45);
#10428=CIRCLE('',#25404,1.5);
#10429=CIRCLE('',#25406,22.45);
#10430=CIRCLE('',#25408,22.45);
#10431=CIRCLE('',#25411,22.45);
#10432=CIRCLE('',#25414,24.55);
#10433=CIRCLE('',#25418,4.01);
#10434=CIRCLE('',#25421,4.01);
#10435=CIRCLE('',#25424,14.7);
#10436=CIRCLE('',#25425,14.3);
#10437=CIRCLE('',#25427,14.7);
#10438=CIRCLE('',#25429,14.3);
#10439=CIRCLE('',#25434,47.);
#10440=CIRCLE('',#25436,11.);
#10734=VERTEX_POINT('',#33459);
#10735=VERTEX_POINT('',#33461);
#10736=VERTEX_POINT('',#33465);
#10737=VERTEX_POINT('',#33468);
#10738=VERTEX_POINT('',#33472);
#10739=VERTEX_POINT('',#33474);
#10740=VERTEX_POINT('',#33478);
#10741=VERTEX_POINT('',#33481);
#10742=VERTEX_POINT('',#33485);
#10743=VERTEX_POINT('',#33487);
#10744=VERTEX_POINT('',#33489);
#10745=VERTEX_POINT('',#33493);
#10746=VERTEX_POINT('',#33497);
#10747=VERTEX_POINT('',#33500);
#10748=VERTEX_POINT('',#33504);
#10749=VERTEX_POINT('',#33505);
#10750=VERTEX_POINT('',#33507);
#10751=VERTEX_POINT('',#33509);
#10752=VERTEX_POINT('',#33536);
#10753=VERTEX_POINT('',#33537);
#10754=VERTEX_POINT('',#33593);
#10755=VERTEX_POINT('',#33598);
#10756=VERTEX_POINT('',#33679);
#10757=VERTEX_POINT('',#33686);
#10758=VERTEX_POINT('',#33695);
#10759=VERTEX_POINT('',#33696);
#10760=VERTEX_POINT('',#33701);
#10761=VERTEX_POINT('',#33702);
#10762=VERTEX_POINT('',#33704);
#10763=VERTEX_POINT('',#33706);
#10764=VERTEX_POINT('',#33708);
#10765=VERTEX_POINT('',#33710);
#10766=VERTEX_POINT('',#33712);
#10767=VERTEX_POINT('',#33714);
#10768=VERTEX_POINT('',#33716);
#10769=VERTEX_POINT('',#33718);
#10770=VERTEX_POINT('',#33721);
#10771=VERTEX_POINT('',#33723);
#10772=VERTEX_POINT('',#33725);
#10773=VERTEX_POINT('',#33727);
#10774=VERTEX_POINT('',#33729);
#10775=VERTEX_POINT('',#33731);
#10776=VERTEX_POINT('',#33733);
#10777=VERTEX_POINT('',#33735);
#10778=VERTEX_POINT('',#33737);
#10779=VERTEX_POINT('',#33739);
#10780=VERTEX_POINT('',#33741);
#10781=VERTEX_POINT('',#33743);
#10782=VERTEX_POINT('',#33745);
#10783=VERTEX_POINT('',#33747);
#10784=VERTEX_POINT('',#33749);
#10785=VERTEX_POINT('',#33751);
#10786=VERTEX_POINT('',#33753);
#10787=VERTEX_POINT('',#33755);
#10788=VERTEX_POINT('',#33757);
#10789=VERTEX_POINT('',#33759);
#10790=VERTEX_POINT('',#33761);
#10791=VERTEX_POINT('',#33763);
#10792=VERTEX_POINT('',#33765);
#10793=VERTEX_POINT('',#33768);
#10794=VERTEX_POINT('',#33769);
#10795=VERTEX_POINT('',#33771);
#10796=VERTEX_POINT('',#33773);
#10797=VERTEX_POINT('',#33775);
#10798=VERTEX_POINT('',#33778);
#10799=VERTEX_POINT('',#33779);
#10800=VERTEX_POINT('',#33781);
#10801=VERTEX_POINT('',#33783);
#10802=VERTEX_POINT('',#33785);
#10803=VERTEX_POINT('',#33788);
#10804=VERTEX_POINT('',#33789);
#10805=VERTEX_POINT('',#33791);
#10806=VERTEX_POINT('',#33793);
#10807=VERTEX_POINT('',#33795);
#10808=VERTEX_POINT('',#33798);
#10809=VERTEX_POINT('',#33801);
#10810=VERTEX_POINT('',#33803);
#10811=VERTEX_POINT('',#33867);
#10812=VERTEX_POINT('',#33894);
#10813=VERTEX_POINT('',#33982);
#10814=VERTEX_POINT('',#33992);
#10815=VERTEX_POINT('',#33996);
#10816=VERTEX_POINT('',#34013);
#10817=VERTEX_POINT('',#34017);
#10818=VERTEX_POINT('',#34021);
#10819=VERTEX_POINT('',#34025);
#10820=VERTEX_POINT('',#34029);
#10821=VERTEX_POINT('',#34033);
#10822=VERTEX_POINT('',#34034);
#10823=VERTEX_POINT('',#34041);
#10824=VERTEX_POINT('',#34043);
#10825=VERTEX_POINT('',#34052);
#10826=VERTEX_POINT('',#34054);
#10827=VERTEX_POINT('',#34056);
#10828=VERTEX_POINT('',#34066);
#10829=VERTEX_POINT('',#34068);
#10830=VERTEX_POINT('',#34070);
#10831=VERTEX_POINT('',#34081);
#10832=VERTEX_POINT('',#34082);
#10833=VERTEX_POINT('',#34089);
#10834=VERTEX_POINT('',#34091);
#10835=VERTEX_POINT('',#34100);
#10836=VERTEX_POINT('',#34102);
#10837=VERTEX_POINT('',#34105);
#10838=VERTEX_POINT('',#34114);
#10839=VERTEX_POINT('',#34116);
#10840=VERTEX_POINT('',#34125);
#10841=VERTEX_POINT('',#34129);
#10842=VERTEX_POINT('',#34136);
#10843=VERTEX_POINT('',#34145);
#10844=VERTEX_POINT('',#34152);
#10845=VERTEX_POINT('',#34161);
#10846=VERTEX_POINT('',#34165);
#10847=VERTEX_POINT('',#34166);
#10848=VERTEX_POINT('',#34168);
#10849=VERTEX_POINT('',#34170);
#10850=VERTEX_POINT('',#34172);
#10851=VERTEX_POINT('',#34174);
#10852=VERTEX_POINT('',#34176);
#10853=VERTEX_POINT('',#34178);
#10854=VERTEX_POINT('',#34181);
#10855=VERTEX_POINT('',#34183);
#10856=VERTEX_POINT('',#34185);
#10857=VERTEX_POINT('',#34187);
#10858=VERTEX_POINT('',#34188);
#10859=VERTEX_POINT('',#34190);
#10860=VERTEX_POINT('',#34192);
#10861=VERTEX_POINT('',#34195);
#10862=VERTEX_POINT('',#34197);
#10863=VERTEX_POINT('',#34199);
#10864=VERTEX_POINT('',#34201);
#10865=VERTEX_POINT('',#34210);
#10866=VERTEX_POINT('',#34214);
#10867=VERTEX_POINT('',#34218);
#10868=VERTEX_POINT('',#34222);
#10869=VERTEX_POINT('',#34249);
#10870=VERTEX_POINT('',#34305);
#10871=VERTEX_POINT('',#34389);
#10872=VERTEX_POINT('',#34396);
#10873=VERTEX_POINT('',#34405);
#10874=VERTEX_POINT('',#34406);
#10875=VERTEX_POINT('',#34411);
#10876=VERTEX_POINT('',#34413);
#10877=VERTEX_POINT('',#34476);
#10878=VERTEX_POINT('',#34503);
#10879=VERTEX_POINT('',#34587);
#10880=VERTEX_POINT('',#34596);
#10881=VERTEX_POINT('',#34600);
#10882=VERTEX_POINT('',#34617);
#10883=VERTEX_POINT('',#34625);
#10884=VERTEX_POINT('',#34626);
#10885=VERTEX_POINT('',#34628);
#10886=VERTEX_POINT('',#34630);
#10887=VERTEX_POINT('',#34634);
#10888=VERTEX_POINT('',#34639);
#10889=VERTEX_POINT('',#34643);
#10890=VERTEX_POINT('',#34644);
#10891=VERTEX_POINT('',#34649);
#10892=VERTEX_POINT('',#34650);
#10893=VERTEX_POINT('',#34657);
#10894=VERTEX_POINT('',#34658);
#10895=VERTEX_POINT('',#34671);
#10896=VERTEX_POINT('',#34673);
#10897=VERTEX_POINT('',#34688);
#10898=VERTEX_POINT('',#34690);
#10899=VERTEX_POINT('',#34694);
#10900=VERTEX_POINT('',#34709);
#10901=VERTEX_POINT('',#34726);
#10902=VERTEX_POINT('',#34743);
#10903=VERTEX_POINT('',#34745);
#10904=VERTEX_POINT('',#34753);
#10905=VERTEX_POINT('',#34755);
#10906=VERTEX_POINT('',#34759);
#10907=VERTEX_POINT('',#34763);
#10908=VERTEX_POINT('',#34767);
#10909=VERTEX_POINT('',#34782);
#10910=VERTEX_POINT('',#34799);
#10911=VERTEX_POINT('',#34816);
#10912=VERTEX_POINT('',#34818);
#10913=VERTEX_POINT('',#34826);
#10914=VERTEX_POINT('',#34828);
#10915=VERTEX_POINT('',#34832);
#10916=VERTEX_POINT('',#34836);
#10917=VERTEX_POINT('',#34869);
#10918=VERTEX_POINT('',#34886);
#10919=VERTEX_POINT('',#34890);
#10920=VERTEX_POINT('',#34905);
#10921=VERTEX_POINT('',#34922);
#10922=VERTEX_POINT('',#34924);
#10923=VERTEX_POINT('',#34928);
#10924=VERTEX_POINT('',#34929);
#10925=VERTEX_POINT('',#34947);
#10926=VERTEX_POINT('',#34964);
#10927=VERTEX_POINT('',#34981);
#10928=VERTEX_POINT('',#34985);
#10929=VERTEX_POINT('',#34989);
#10930=VERTEX_POINT('',#34995);
#10931=VERTEX_POINT('',#34999);
#10932=VERTEX_POINT('',#35003);
#10933=VERTEX_POINT('',#35007);
#10934=VERTEX_POINT('',#35011);
#10935=VERTEX_POINT('',#35015);
#10936=VERTEX_POINT('',#35019);
#10937=VERTEX_POINT('',#35023);
#10938=VERTEX_POINT('',#35025);
#10939=VERTEX_POINT('',#35029);
#10940=VERTEX_POINT('',#35033);
#10941=VERTEX_POINT('',#35037);
#10942=VERTEX_POINT('',#35041);
#10943=VERTEX_POINT('',#35045);
#10944=VERTEX_POINT('',#35051);
#10945=VERTEX_POINT('',#35057);
#10946=VERTEX_POINT('',#35059);
#10947=VERTEX_POINT('',#35063);
#10948=VERTEX_POINT('',#35067);
#10949=VERTEX_POINT('',#35071);
#10950=VERTEX_POINT('',#35075);
#10951=VERTEX_POINT('',#35087);
#10952=VERTEX_POINT('',#35104);
#10953=VERTEX_POINT('',#35123);
#10954=VERTEX_POINT('',#35127);
#10955=VERTEX_POINT('',#35144);
#10956=VERTEX_POINT('',#35148);
#10957=VERTEX_POINT('',#35154);
#10958=VERTEX_POINT('',#35156);
#10959=VERTEX_POINT('',#35192);
#10960=VERTEX_POINT('',#35207);
#10961=VERTEX_POINT('',#35209);
#10962=VERTEX_POINT('',#35213);
#10963=VERTEX_POINT('',#35217);
#10964=VERTEX_POINT('',#35223);
#10965=VERTEX_POINT('',#35225);
#10966=VERTEX_POINT('',#35229);
#10967=VERTEX_POINT('',#35233);
#10968=VERTEX_POINT('',#35235);
#10969=VERTEX_POINT('',#35239);
#10970=VERTEX_POINT('',#35243);
#10971=VERTEX_POINT('',#35249);
#10972=VERTEX_POINT('',#35251);
#10973=VERTEX_POINT('',#35255);
#10974=VERTEX_POINT('',#35259);
#10975=VERTEX_POINT('',#35265);
#10976=VERTEX_POINT('',#35272);
#10977=VERTEX_POINT('',#35277);
#10978=VERTEX_POINT('',#35282);
#10979=VERTEX_POINT('',#35284);
#10980=VERTEX_POINT('',#35287);
#10981=VERTEX_POINT('',#35291);
#10982=VERTEX_POINT('',#35299);
#10983=VERTEX_POINT('',#35303);
#13017=EDGE_CURVE('',#10734,#10734,#10272,.T.);
#13018=EDGE_CURVE('',#10734,#10735,#4534,.T.);
#13019=EDGE_CURVE('',#10735,#10735,#10273,.T.);
#13020=EDGE_CURVE('',#10736,#10736,#10274,.T.);
#13021=EDGE_CURVE('',#10735,#10737,#4535,.T.);
#13022=EDGE_CURVE('',#10737,#10737,#10275,.T.);
#13023=EDGE_CURVE('',#10738,#10738,#10276,.T.);
#13024=EDGE_CURVE('',#10738,#10739,#4536,.T.);
#13025=EDGE_CURVE('',#10739,#10739,#10277,.T.);
#13026=EDGE_CURVE('',#10740,#10740,#10278,.T.);
#13027=EDGE_CURVE('',#10739,#10741,#4537,.T.);
#13028=EDGE_CURVE('',#10741,#10741,#10279,.T.);
#13029=EDGE_CURVE('',#10742,#10742,#10280,.T.);
#13030=EDGE_CURVE('',#10742,#10743,#4538,.T.);
#13031=EDGE_CURVE('',#10743,#10744,#10281,.T.);
#13032=EDGE_CURVE('',#10744,#10743,#10282,.T.);
#13033=EDGE_CURVE('',#10744,#10745,#4539,.T.);
#13034=EDGE_CURVE('',#10745,#10745,#10283,.T.);
#13035=EDGE_CURVE('',#10746,#10746,#10284,.T.);
#13036=EDGE_CURVE('',#10747,#10747,#10285,.T.);
#13037=EDGE_CURVE('',#10747,#10745,#4540,.T.);
#13038=EDGE_CURVE('',#10748,#10749,#4541,.T.);
#13039=EDGE_CURVE('',#10750,#10748,#10286,.T.);
#13040=EDGE_CURVE('',#10751,#10750,#4542,.T.);
#13041=EDGE_CURVE('',#10749,#10751,#10287,.T.);
#13042=EDGE_CURVE('',#10752,#10753,#235,.T.);
#13043=EDGE_CURVE('',#10754,#10753,#236,.T.);
#13044=EDGE_CURVE('',#10754,#10755,#237,.T.);
#13045=EDGE_CURVE('',#10755,#10752,#4543,.T.);
#13046=EDGE_CURVE('',#10753,#10756,#238,.T.);
#13047=EDGE_CURVE('',#10756,#10757,#4544,.T.);
#13048=EDGE_CURVE('',#10757,#10754,#239,.T.);
#13049=EDGE_CURVE('',#10758,#10759,#4545,.F.);
#13050=EDGE_CURVE('',#10759,#10757,#4546,.T.);
#13051=EDGE_CURVE('',#10756,#10758,#4547,.T.);
#13052=EDGE_CURVE('',#10760,#10761,#4548,.T.);
#13053=EDGE_CURVE('',#10762,#10760,#10288,.T.);
#13054=EDGE_CURVE('',#10763,#10762,#4549,.T.);
#13055=EDGE_CURVE('',#10764,#10763,#10289,.T.);
#13056=EDGE_CURVE('',#10765,#10764,#4550,.T.);
#13057=EDGE_CURVE('',#10766,#10765,#10290,.T.);
#13058=EDGE_CURVE('',#10767,#10766,#4551,.T.);
#13059=EDGE_CURVE('',#10768,#10767,#10291,.T.);
#13060=EDGE_CURVE('',#10769,#10768,#4552,.T.);
#13061=EDGE_CURVE('',#10761,#10769,#10292,.T.);
#13062=EDGE_CURVE('',#10770,#10770,#10293,.T.);
#13063=EDGE_CURVE('',#10771,#10755,#4553,.T.);
#13064=EDGE_CURVE('',#10772,#10771,#4554,.T.);
#13065=EDGE_CURVE('',#10773,#10772,#4555,.T.);
#13066=EDGE_CURVE('',#10774,#10773,#10294,.T.);
#13067=EDGE_CURVE('',#10775,#10774,#4556,.T.);
#13068=EDGE_CURVE('',#10776,#10775,#4557,.T.);
#13069=EDGE_CURVE('',#10777,#10776,#4558,.T.);
#13070=EDGE_CURVE('',#10778,#10777,#10295,.T.);
#13071=EDGE_CURVE('',#10779,#10778,#10296,.T.);
#13072=EDGE_CURVE('',#10780,#10779,#4559,.T.);
#13073=EDGE_CURVE('',#10781,#10780,#10297,.T.);
#13074=EDGE_CURVE('',#10782,#10781,#4560,.T.);
#13075=EDGE_CURVE('',#10783,#10782,#10298,.T.);
#13076=EDGE_CURVE('',#10784,#10783,#4561,.T.);
#13077=EDGE_CURVE('',#10785,#10784,#10299,.T.);
#13078=EDGE_CURVE('',#10786,#10785,#10300,.T.);
#13079=EDGE_CURVE('',#10787,#10786,#4562,.T.);
#13080=EDGE_CURVE('',#10788,#10787,#4563,.T.);
#13081=EDGE_CURVE('',#10789,#10788,#4564,.T.);
#13082=EDGE_CURVE('',#10790,#10789,#4565,.T.);
#13083=EDGE_CURVE('',#10791,#10790,#4566,.T.);
#13084=EDGE_CURVE('',#10792,#10791,#10301,.T.);
#13085=EDGE_CURVE('',#10752,#10792,#4567,.T.);
#13086=EDGE_CURVE('',#10793,#10794,#10302,.T.);
#13087=EDGE_CURVE('',#10795,#10793,#4568,.T.);
#13088=EDGE_CURVE('',#10796,#10795,#10303,.T.);
#13089=EDGE_CURVE('',#10797,#10796,#10304,.T.);
#13090=EDGE_CURVE('',#10794,#10797,#4569,.T.);
#13091=EDGE_CURVE('',#10798,#10799,#10305,.T.);
#13092=EDGE_CURVE('',#10798,#10800,#10306,.T.);
#13093=EDGE_CURVE('',#10800,#10801,#10307,.T.);
#13094=EDGE_CURVE('',#10802,#10801,#10308,.T.);
#13095=EDGE_CURVE('',#10802,#10799,#10309,.T.);
#13096=EDGE_CURVE('',#10803,#10804,#10310,.T.);
#13097=EDGE_CURVE('',#10805,#10803,#4570,.T.);
#13098=EDGE_CURVE('',#10806,#10805,#10311,.T.);
#13099=EDGE_CURVE('',#10807,#10806,#10312,.T.);
#13100=EDGE_CURVE('',#10804,#10807,#4571,.T.);
#13101=EDGE_CURVE('',#10808,#10808,#10313,.T.);
#13102=EDGE_CURVE('',#10757,#10809,#4572,.T.);
#13103=EDGE_CURVE('',#10810,#10809,#240,.T.);
#13104=EDGE_CURVE('',#10771,#10810,#241,.T.);
#13105=EDGE_CURVE('',#10811,#10759,#4573,.T.);
#13106=EDGE_CURVE('',#10809,#10811,#4574,.T.);
#13107=EDGE_CURVE('',#10812,#10810,#242,.T.);
#13108=EDGE_CURVE('',#10812,#10772,#243,.T.);
#13109=EDGE_CURVE('',#10809,#10813,#4575,.T.);
#13110=EDGE_CURVE('',#10813,#10812,#244,.T.);
#13111=EDGE_CURVE('',#10811,#10814,#4576,.F.);
#13112=EDGE_CURVE('',#10814,#10813,#4577,.T.);
#13113=EDGE_CURVE('',#10813,#10815,#4578,.T.);
#13114=EDGE_CURVE('',#10773,#10815,#245,.F.);
#13115=EDGE_CURVE('',#10816,#10814,#4579,.T.);
#13116=EDGE_CURVE('',#10815,#10816,#4580,.T.);
#13117=EDGE_CURVE('',#10740,#10817,#4581,.T.);
#13118=EDGE_CURVE('',#10817,#10817,#10314,.T.);
#13119=EDGE_CURVE('',#10818,#10818,#10315,.T.);
#13120=EDGE_CURVE('',#10818,#10817,#4582,.T.);
#13121=EDGE_CURVE('',#10736,#10819,#4583,.T.);
#13122=EDGE_CURVE('',#10819,#10819,#10316,.T.);
#13123=EDGE_CURVE('',#10820,#10820,#10317,.T.);
#13124=EDGE_CURVE('',#10820,#10819,#4584,.T.);
#13125=EDGE_CURVE('',#10821,#10822,#246,.F.);
#13126=EDGE_CURVE('',#10822,#10823,#4585,.T.);
#13127=EDGE_CURVE('',#10823,#10824,#247,.F.);
#13128=EDGE_CURVE('',#10824,#10821,#4586,.T.);
#13129=EDGE_CURVE('',#10825,#10825,#10318,.T.);
#13130=EDGE_CURVE('',#10825,#10826,#4587,.T.);
#13131=EDGE_CURVE('',#10826,#10827,#10319,.T.);
#13132=EDGE_CURVE('',#10823,#10827,#248,.F.);
#13133=EDGE_CURVE('',#10828,#10822,#10320,.T.);
#13134=EDGE_CURVE('',#10829,#10828,#4588,.T.);
#13135=EDGE_CURVE('',#10830,#10829,#249,.F.);
#13136=EDGE_CURVE('',#10830,#10826,#10321,.T.);
#13137=EDGE_CURVE('',#10831,#10832,#250,.F.);
#13138=EDGE_CURVE('',#10832,#10833,#4589,.T.);
#13139=EDGE_CURVE('',#10833,#10834,#251,.F.);
#13140=EDGE_CURVE('',#10834,#10831,#4590,.T.);
#13141=EDGE_CURVE('',#10835,#10835,#10322,.T.);
#13142=EDGE_CURVE('',#10835,#10836,#4591,.T.);
#13143=EDGE_CURVE('',#10833,#10836,#10323,.T.);
#13144=EDGE_CURVE('',#10837,#10832,#252,.F.);
#13145=EDGE_CURVE('',#10837,#10838,#10324,.T.);
#13146=EDGE_CURVE('',#10839,#10838,#253,.F.);
#13147=EDGE_CURVE('',#10840,#10839,#4592,.T.);
#13148=EDGE_CURVE('',#10836,#10840,#10325,.T.);
#13149=EDGE_CURVE('',#10841,#10840,#254,.F.);
#13150=EDGE_CURVE('',#10839,#10842,#255,.F.);
#13151=EDGE_CURVE('',#10842,#10841,#4593,.T.);
#13152=EDGE_CURVE('',#10843,#10829,#256,.F.);
#13153=EDGE_CURVE('',#10828,#10844,#257,.F.);
#13154=EDGE_CURVE('',#10844,#10843,#4594,.T.);
#13155=EDGE_CURVE('',#10845,#10845,#10326,.T.);
#13156=EDGE_CURVE('',#10845,#10820,#4595,.T.);
#13157=EDGE_CURVE('',#10846,#10847,#10327,.T.);
#13158=EDGE_CURVE('',#10848,#10846,#4596,.T.);
#13159=EDGE_CURVE('',#10849,#10848,#10328,.T.);
#13160=EDGE_CURVE('',#10850,#10849,#4597,.T.);
#13161=EDGE_CURVE('',#10851,#10850,#10329,.T.);
#13162=EDGE_CURVE('',#10852,#10851,#4598,.T.);
#13163=EDGE_CURVE('',#10853,#10852,#10330,.T.);
#13164=EDGE_CURVE('',#10847,#10853,#4599,.T.);
#13165=EDGE_CURVE('',#10854,#10854,#10331,.T.);
#13166=EDGE_CURVE('',#10855,#10855,#10332,.T.);
#13167=EDGE_CURVE('',#10856,#10856,#10333,.T.);
#13168=EDGE_CURVE('',#10857,#10858,#4600,.T.);
#13169=EDGE_CURVE('',#10859,#10857,#10334,.T.);
#13170=EDGE_CURVE('',#10860,#10859,#4601,.T.);
#13171=EDGE_CURVE('',#10858,#10860,#10335,.T.);
#13172=EDGE_CURVE('',#10861,#10861,#10336,.T.);
#13173=EDGE_CURVE('',#10862,#10862,#10337,.T.);
#13174=EDGE_CURVE('',#10863,#10863,#10338,.T.);
#13175=EDGE_CURVE('',#10864,#10864,#10339,.T.);
#13176=EDGE_CURVE('',#10854,#10835,#4602,.T.);
#13177=EDGE_CURVE('',#10864,#10825,#4603,.T.);
#13178=EDGE_CURVE('',#10855,#10818,#4604,.T.);
#13179=EDGE_CURVE('',#10863,#10865,#4605,.T.);
#13180=EDGE_CURVE('',#10865,#10865,#10340,.T.);
#13181=EDGE_CURVE('',#10866,#10866,#10341,.T.);
#13182=EDGE_CURVE('',#10866,#10865,#4606,.T.);
#13183=EDGE_CURVE('',#10856,#10867,#4607,.T.);
#13184=EDGE_CURVE('',#10867,#10867,#10342,.T.);
#13185=EDGE_CURVE('',#10868,#10868,#10343,.T.);
#13186=EDGE_CURVE('',#10868,#10867,#4608,.T.);
#13187=EDGE_CURVE('',#10787,#10869,#258,.T.);
#13188=EDGE_CURVE('',#10870,#10869,#259,.T.);
#13189=EDGE_CURVE('',#10870,#10788,#260,.T.);
#13190=EDGE_CURVE('',#10869,#10871,#261,.T.);
#13191=EDGE_CURVE('',#10871,#10872,#4609,.T.);
#13192=EDGE_CURVE('',#10872,#10870,#262,.T.);
#13193=EDGE_CURVE('',#10873,#10874,#4610,.F.);
#13194=EDGE_CURVE('',#10874,#10872,#4611,.T.);
#13195=EDGE_CURVE('',#10871,#10873,#4612,.T.);
#13196=EDGE_CURVE('',#10872,#10875,#4613,.T.);
#13197=EDGE_CURVE('',#10876,#10875,#263,.T.);
#13198=EDGE_CURVE('',#10789,#10876,#264,.T.);
#13199=EDGE_CURVE('',#10877,#10874,#4614,.T.);
#13200=EDGE_CURVE('',#10875,#10877,#4615,.T.);
#13201=EDGE_CURVE('',#10878,#10876,#265,.T.);
#13202=EDGE_CURVE('',#10878,#10790,#266,.T.);
#13203=EDGE_CURVE('',#10875,#10879,#4616,.T.);
#13204=EDGE_CURVE('',#10879,#10878,#267,.T.);
#13205=EDGE_CURVE('',#10877,#10880,#4617,.F.);
#13206=EDGE_CURVE('',#10880,#10879,#4618,.T.);
#13207=EDGE_CURVE('',#10879,#10881,#4619,.T.);
#13208=EDGE_CURVE('',#10791,#10881,#268,.T.);
#13209=EDGE_CURVE('',#10882,#10880,#4620,.T.);
#13210=EDGE_CURVE('',#10881,#10882,#4621,.T.);
#13211=EDGE_CURVE('',#10808,#10868,#4622,.T.);
#13212=EDGE_CURVE('',#10770,#10866,#4623,.T.);
#13213=EDGE_CURVE('',#10883,#10884,#4624,.F.);
#13214=EDGE_CURVE('',#10884,#10885,#4625,.T.);
#13215=EDGE_CURVE('',#10885,#10886,#4626,.T.);
#13216=EDGE_CURVE('',#10886,#10883,#4627,.T.);
#13217=EDGE_CURVE('',#10887,#10775,#4628,.T.);
#13218=EDGE_CURVE('',#10775,#10886,#10344,.T.);
#13219=EDGE_CURVE('',#10885,#10887,#10345,.T.);
#13220=EDGE_CURVE('',#10888,#10776,#4629,.T.);
#13221=EDGE_CURVE('',#10887,#10888,#4630,.T.);
#13222=EDGE_CURVE('',#10889,#10890,#4631,.T.);
#13223=EDGE_CURVE('',#10890,#10776,#10346,.T.);
#13224=EDGE_CURVE('',#10888,#10889,#10347,.T.);
#13225=EDGE_CURVE('',#10891,#10892,#4632,.F.);
#13226=EDGE_CURVE('',#10892,#10890,#4633,.T.);
#13227=EDGE_CURVE('',#10889,#10891,#4634,.T.);
#13228=EDGE_CURVE('',#10891,#10884,#4635,.T.);
#13229=EDGE_CURVE('',#10893,#10894,#269,.F.);
#13230=EDGE_CURVE('',#10894,#10895,#10348,.T.);
#13231=EDGE_CURVE('',#10895,#10896,#270,.F.);
#13232=EDGE_CURVE('',#10896,#10893,#10349,.T.);
#13233=EDGE_CURVE('',#10897,#10894,#4636,.T.);
#13234=EDGE_CURVE('',#10898,#10897,#10350,.T.);
#13235=EDGE_CURVE('',#10895,#10898,#4637,.T.);
#13236=EDGE_CURVE('',#10806,#10899,#271,.T.);
#13237=EDGE_CURVE('',#10899,#10900,#10351,.T.);
#13238=EDGE_CURVE('',#10807,#10900,#272,.T.);
#13239=EDGE_CURVE('',#10805,#10901,#273,.T.);
#13240=EDGE_CURVE('',#10901,#10899,#10352,.T.);
#13241=EDGE_CURVE('',#10804,#10902,#10353,.T.);
#13242=EDGE_CURVE('',#10902,#10903,#10354,.T.);
#13243=EDGE_CURVE('',#10903,#10803,#10355,.T.);
#13244=EDGE_CURVE('',#10903,#10901,#4638,.T.);
#13245=EDGE_CURVE('',#10900,#10902,#4639,.T.);
#13246=EDGE_CURVE('',#10904,#10901,#4640,.T.);
#13247=EDGE_CURVE('',#10905,#10904,#10356,.T.);
#13248=EDGE_CURVE('',#10905,#10899,#4641,.T.);
#13249=EDGE_CURVE('',#10903,#10906,#4642,.T.);
#13250=EDGE_CURVE('',#10906,#10904,#4643,.T.);
#13251=EDGE_CURVE('',#10902,#10907,#4644,.T.);
#13252=EDGE_CURVE('',#10907,#10906,#10357,.T.);
#13253=EDGE_CURVE('',#10796,#10908,#274,.T.);
#13254=EDGE_CURVE('',#10908,#10909,#10358,.T.);
#13255=EDGE_CURVE('',#10797,#10909,#275,.T.);
#13256=EDGE_CURVE('',#10795,#10910,#276,.T.);
#13257=EDGE_CURVE('',#10910,#10908,#10359,.T.);
#13258=EDGE_CURVE('',#10794,#10911,#10360,.T.);
#13259=EDGE_CURVE('',#10911,#10912,#10361,.T.);
#13260=EDGE_CURVE('',#10912,#10793,#10362,.T.);
#13261=EDGE_CURVE('',#10912,#10910,#4645,.T.);
#13262=EDGE_CURVE('',#10909,#10911,#4646,.T.);
#13263=EDGE_CURVE('',#10913,#10910,#4647,.T.);
#13264=EDGE_CURVE('',#10914,#10913,#10363,.T.);
#13265=EDGE_CURVE('',#10914,#10908,#4648,.T.);
#13266=EDGE_CURVE('',#10912,#10915,#4649,.T.);
#13267=EDGE_CURVE('',#10915,#10913,#4650,.T.);
#13268=EDGE_CURVE('',#10911,#10916,#4651,.T.);
#13269=EDGE_CURVE('',#10916,#10915,#10364,.T.);
#13270=EDGE_CURVE('',#10769,#10898,#277,.F.);
#13271=EDGE_CURVE('',#10897,#10761,#278,.F.);
#13272=EDGE_CURVE('',#10815,#10917,#10365,.T.);
#13273=EDGE_CURVE('',#10917,#10774,#279,.F.);
#13274=EDGE_CURVE('',#10918,#10816,#10366,.T.);
#13275=EDGE_CURVE('',#10918,#10917,#4652,.T.);
#13276=EDGE_CURVE('',#10784,#10919,#280,.F.);
#13277=EDGE_CURVE('',#10919,#10920,#10367,.T.);
#13278=EDGE_CURVE('',#10920,#10785,#281,.F.);
#13279=EDGE_CURVE('',#10921,#10919,#4653,.T.);
#13280=EDGE_CURVE('',#10922,#10921,#10368,.T.);
#13281=EDGE_CURVE('',#10922,#10920,#4654,.T.);
#13282=EDGE_CURVE('',#10923,#10924,#4655,.T.);
#13283=EDGE_CURVE('',#10924,#10780,#10369,.T.);
#13284=EDGE_CURVE('',#10779,#10923,#282,.T.);
#13285=EDGE_CURVE('',#10778,#10925,#283,.T.);
#13286=EDGE_CURVE('',#10925,#10923,#10370,.T.);
#13287=EDGE_CURVE('',#10777,#10926,#284,.F.);
#13288=EDGE_CURVE('',#10926,#10925,#10371,.T.);
#13289=EDGE_CURVE('',#10927,#10781,#10372,.T.);
#13290=EDGE_CURVE('',#10924,#10927,#10373,.T.);
#13291=EDGE_CURVE('',#10928,#10782,#10374,.T.);
#13292=EDGE_CURVE('',#10927,#10928,#4656,.T.);
#13293=EDGE_CURVE('',#10929,#10783,#10375,.T.);
#13294=EDGE_CURVE('',#10928,#10929,#10376,.T.);
#13295=EDGE_CURVE('',#10929,#10919,#4657,.T.);
#13296=EDGE_CURVE('',#10929,#10930,#4658,.T.);
#13297=EDGE_CURVE('',#10930,#10921,#4659,.T.);
#13298=EDGE_CURVE('',#10928,#10931,#4660,.T.);
#13299=EDGE_CURVE('',#10931,#10930,#10377,.T.);
#13300=EDGE_CURVE('',#10927,#10932,#4661,.T.);
#13301=EDGE_CURVE('',#10932,#10931,#4662,.T.);
#13302=EDGE_CURVE('',#10924,#10933,#4663,.T.);
#13303=EDGE_CURVE('',#10933,#10932,#10378,.T.);
#13304=EDGE_CURVE('',#10923,#10934,#4664,.T.);
#13305=EDGE_CURVE('',#10934,#10933,#4665,.T.);
#13306=EDGE_CURVE('',#10935,#10925,#4666,.T.);
#13307=EDGE_CURVE('',#10934,#10935,#10379,.T.);
#13308=EDGE_CURVE('',#10926,#10936,#4667,.T.);
#13309=EDGE_CURVE('',#10935,#10936,#10380,.T.);
#13310=EDGE_CURVE('',#10762,#10937,#10381,.T.);
#13311=EDGE_CURVE('',#10937,#10938,#4668,.T.);
#13312=EDGE_CURVE('',#10938,#10763,#10382,.T.);
#13313=EDGE_CURVE('',#10939,#10764,#10383,.T.);
#13314=EDGE_CURVE('',#10938,#10939,#10384,.T.);
#13315=EDGE_CURVE('',#10940,#10765,#10385,.T.);
#13316=EDGE_CURVE('',#10939,#10940,#4669,.T.);
#13317=EDGE_CURVE('',#10941,#10766,#10386,.T.);
#13318=EDGE_CURVE('',#10940,#10941,#10387,.T.);
#13319=EDGE_CURVE('',#10942,#10767,#10388,.T.);
#13320=EDGE_CURVE('',#10941,#10942,#4670,.T.);
#13321=EDGE_CURVE('',#10943,#10768,#10389,.T.);
#13322=EDGE_CURVE('',#10942,#10943,#10390,.T.);
#13323=EDGE_CURVE('',#10943,#10898,#4671,.T.);
#13324=EDGE_CURVE('',#10760,#10944,#10391,.T.);
#13325=EDGE_CURVE('',#10944,#10937,#10392,.T.);
#13326=EDGE_CURVE('',#10897,#10944,#4672,.T.);
#13327=EDGE_CURVE('',#10940,#10945,#4673,.T.);
#13328=EDGE_CURVE('',#10946,#10945,#10393,.T.);
#13329=EDGE_CURVE('',#10941,#10946,#4674,.T.);
#13330=EDGE_CURVE('',#10939,#10947,#4675,.T.);
#13331=EDGE_CURVE('',#10945,#10947,#4676,.T.);
#13332=EDGE_CURVE('',#10938,#10948,#4677,.T.);
#13333=EDGE_CURVE('',#10947,#10948,#10394,.T.);
#13334=EDGE_CURVE('',#10937,#10949,#4678,.T.);
#13335=EDGE_CURVE('',#10948,#10949,#4679,.T.);
#13336=EDGE_CURVE('',#10944,#10950,#4680,.T.);
#13337=EDGE_CURVE('',#10949,#10950,#10395,.T.);
#13338=EDGE_CURVE('',#10890,#10926,#4681,.T.);
#13339=EDGE_CURVE('',#10936,#10892,#4682,.T.);
#13340=EDGE_CURVE('',#10917,#10886,#4683,.T.);
#13341=EDGE_CURVE('',#10883,#10918,#4684,.T.);
#13342=EDGE_CURVE('',#10881,#10951,#10396,.T.);
#13343=EDGE_CURVE('',#10951,#10792,#285,.F.);
#13344=EDGE_CURVE('',#10786,#10952,#286,.T.);
#13345=EDGE_CURVE('',#10952,#10871,#4685,.T.);
#13346=EDGE_CURVE('',#10920,#10952,#10397,.T.);
#13347=EDGE_CURVE('',#10953,#10882,#10398,.T.);
#13348=EDGE_CURVE('',#10953,#10951,#4686,.T.);
#13349=EDGE_CURVE('',#10954,#10952,#4687,.T.);
#13350=EDGE_CURVE('',#10873,#10954,#4688,.T.);
#13351=EDGE_CURVE('',#10954,#10922,#10399,.T.);
#13352=EDGE_CURVE('',#10847,#10946,#10400,.T.);
#13353=EDGE_CURVE('',#10945,#10846,#10401,.T.);
#13354=EDGE_CURVE('',#10947,#10848,#10402,.T.);
#13355=EDGE_CURVE('',#10948,#10849,#10403,.T.);
#13356=EDGE_CURVE('',#10949,#10850,#10404,.T.);
#13357=EDGE_CURVE('',#10950,#10851,#10405,.T.);
#13358=EDGE_CURVE('',#10955,#10852,#10406,.T.);
#13359=EDGE_CURVE('',#10950,#10955,#4689,.T.);
#13360=EDGE_CURVE('',#10956,#10853,#10407,.T.);
#13361=EDGE_CURVE('',#10955,#10956,#10408,.T.);
#13362=EDGE_CURVE('',#10956,#10946,#4690,.T.);
#13363=EDGE_CURVE('',#10957,#10957,#10409,.T.);
#13364=EDGE_CURVE('',#10957,#10958,#10410,.T.);
#13365=EDGE_CURVE('',#10958,#10958,#10411,.T.);
#13366=EDGE_CURVE('',#10843,#10824,#10412,.T.);
#13367=EDGE_CURVE('',#10799,#10844,#287,.F.);
#13368=EDGE_CURVE('',#10841,#10802,#288,.F.);
#13369=EDGE_CURVE('',#10831,#10842,#10413,.T.);
#13370=EDGE_CURVE('',#10801,#10834,#289,.F.);
#13371=EDGE_CURVE('',#10800,#10957,#4691,.T.);
#13372=EDGE_CURVE('',#10821,#10798,#290,.F.);
#13373=EDGE_CURVE('',#10959,#10959,#10414,.T.);
#13374=EDGE_CURVE('',#10951,#10756,#4692,.T.);
#13375=EDGE_CURVE('',#10758,#10953,#4693,.T.);
#13376=EDGE_CURVE('',#10827,#10830,#10415,.T.);
#13377=EDGE_CURVE('',#10838,#10837,#10416,.T.);
#13378=EDGE_CURVE('',#10858,#10960,#10417,.T.);
#13379=EDGE_CURVE('',#10960,#10961,#4694,.T.);
#13380=EDGE_CURVE('',#10961,#10857,#10418,.T.);
#13381=EDGE_CURVE('',#10962,#10859,#10419,.T.);
#13382=EDGE_CURVE('',#10961,#10962,#10420,.T.);
#13383=EDGE_CURVE('',#10963,#10860,#10421,.T.);
#13384=EDGE_CURVE('',#10962,#10963,#4695,.T.);
#13385=EDGE_CURVE('',#10963,#10960,#10422,.T.);
#13386=EDGE_CURVE('',#10961,#10964,#4696,.T.);
#13387=EDGE_CURVE('',#10964,#10965,#10423,.T.);
#13388=EDGE_CURVE('',#10962,#10965,#4697,.T.);
#13389=EDGE_CURVE('',#10960,#10966,#4698,.T.);
#13390=EDGE_CURVE('',#10966,#10964,#4699,.T.);
#13391=EDGE_CURVE('',#10749,#10967,#10424,.T.);
#13392=EDGE_CURVE('',#10967,#10968,#4700,.T.);
#13393=EDGE_CURVE('',#10968,#10748,#10425,.T.);
#13394=EDGE_CURVE('',#10969,#10750,#10426,.T.);
#13395=EDGE_CURVE('',#10968,#10969,#10427,.T.);
#13396=EDGE_CURVE('',#10970,#10751,#10428,.T.);
#13397=EDGE_CURVE('',#10969,#10970,#4701,.T.);
#13398=EDGE_CURVE('',#10970,#10967,#10429,.T.);
#13399=EDGE_CURVE('',#10968,#10971,#4702,.T.);
#13400=EDGE_CURVE('',#10971,#10972,#10430,.T.);
#13401=EDGE_CURVE('',#10969,#10972,#4703,.T.);
#13402=EDGE_CURVE('',#10967,#10973,#4704,.T.);
#13403=EDGE_CURVE('',#10973,#10971,#4705,.T.);
#13404=EDGE_CURVE('',#10970,#10974,#4706,.T.);
#13405=EDGE_CURVE('',#10974,#10973,#10431,.T.);
#13406=EDGE_CURVE('',#10972,#10974,#4707,.T.);
#13407=EDGE_CURVE('',#10963,#10975,#4708,.T.);
#13408=EDGE_CURVE('',#10975,#10966,#10432,.T.);
#13409=EDGE_CURVE('',#10965,#10975,#4709,.T.);
#13410=EDGE_CURVE('',#10861,#10976,#4710,.T.);
#13411=EDGE_CURVE('',#10976,#10976,#10433,.T.);
#13412=EDGE_CURVE('',#10862,#10977,#4711,.T.);
#13413=EDGE_CURVE('',#10977,#10977,#10434,.T.);
#13414=EDGE_CURVE('',#10978,#10978,#10435,.T.);
#13415=EDGE_CURVE('',#10979,#10979,#10436,.T.);
#13416=EDGE_CURVE('',#10978,#10980,#4712,.T.);
#13417=EDGE_CURVE('',#10980,#10980,#10437,.T.);
#13418=EDGE_CURVE('',#10981,#10981,#10438,.T.);
#13419=EDGE_CURVE('',#10981,#10746,#4713,.T.);
#13420=EDGE_CURVE('',#10959,#10979,#4714,.T.);
#13421=EDGE_CURVE('',#10982,#10914,#10439,.T.);
#13422=EDGE_CURVE('',#10909,#10982,#4715,.T.);
#13423=EDGE_CURVE('',#10983,#10905,#10440,.T.);
#13424=EDGE_CURVE('',#10900,#10983,#4716,.T.);
#13425=EDGE_CURVE('',#10893,#10896,#4717,.T.);
#13426=EDGE_CURVE('',#10943,#10955,#4718,.T.);
#13427=EDGE_CURVE('',#10983,#10907,#4719,.T.);
#13428=EDGE_CURVE('',#10982,#10916,#4720,.T.);
#13429=EDGE_CURVE('',#10942,#10956,#4721,.T.);
#16528=ORIENTED_EDGE('',*,*,#13017,.T.);
#16529=ORIENTED_EDGE('',*,*,#13018,.T.);
#16530=ORIENTED_EDGE('',*,*,#13019,.T.);
#16531=ORIENTED_EDGE('',*,*,#13018,.F.);
#16532=ORIENTED_EDGE('',*,*,#13017,.F.);
#16533=ORIENTED_EDGE('',*,*,#13020,.F.);
#16534=ORIENTED_EDGE('',*,*,#13019,.F.);
#16535=ORIENTED_EDGE('',*,*,#13021,.T.);
#16536=ORIENTED_EDGE('',*,*,#13022,.F.);
#16537=ORIENTED_EDGE('',*,*,#13021,.F.);
#16538=ORIENTED_EDGE('',*,*,#13023,.T.);
#16539=ORIENTED_EDGE('',*,*,#13024,.T.);
#16540=ORIENTED_EDGE('',*,*,#13025,.T.);
#16541=ORIENTED_EDGE('',*,*,#13024,.F.);
#16542=ORIENTED_EDGE('',*,*,#13023,.F.);
#16543=ORIENTED_EDGE('',*,*,#13026,.F.);
#16544=ORIENTED_EDGE('',*,*,#13025,.F.);
#16545=ORIENTED_EDGE('',*,*,#13027,.T.);
#16546=ORIENTED_EDGE('',*,*,#13028,.F.);
#16547=ORIENTED_EDGE('',*,*,#13027,.F.);
#16548=ORIENTED_EDGE('',*,*,#13029,.T.);
#16549=ORIENTED_EDGE('',*,*,#13030,.T.);
#16550=ORIENTED_EDGE('',*,*,#13031,.T.);
#16551=ORIENTED_EDGE('',*,*,#13032,.T.);
#16552=ORIENTED_EDGE('',*,*,#13030,.F.);
#16553=ORIENTED_EDGE('',*,*,#13031,.F.);
#16554=ORIENTED_EDGE('',*,*,#13032,.F.);
#16555=ORIENTED_EDGE('',*,*,#13033,.T.);
#16556=ORIENTED_EDGE('',*,*,#13034,.F.);
#16557=ORIENTED_EDGE('',*,*,#13033,.F.);
#16558=ORIENTED_EDGE('',*,*,#13035,.F.);
#16559=ORIENTED_EDGE('',*,*,#13029,.F.);
#16560=ORIENTED_EDGE('',*,*,#13036,.T.);
#16561=ORIENTED_EDGE('',*,*,#13037,.T.);
#16562=ORIENTED_EDGE('',*,*,#13034,.T.);
#16563=ORIENTED_EDGE('',*,*,#13037,.F.);
#16564=ORIENTED_EDGE('',*,*,#13038,.F.);
#16565=ORIENTED_EDGE('',*,*,#13039,.F.);
#16566=ORIENTED_EDGE('',*,*,#13040,.F.);
#16567=ORIENTED_EDGE('',*,*,#13041,.F.);
#16568=ORIENTED_EDGE('',*,*,#13036,.F.);
#16569=ORIENTED_EDGE('',*,*,#13042,.T.);
#16570=ORIENTED_EDGE('',*,*,#13043,.F.);
#16571=ORIENTED_EDGE('',*,*,#13044,.T.);
#16572=ORIENTED_EDGE('',*,*,#13045,.T.);
#16573=ORIENTED_EDGE('',*,*,#13043,.T.);
#16574=ORIENTED_EDGE('',*,*,#13046,.T.);
#16575=ORIENTED_EDGE('',*,*,#13047,.T.);
#16576=ORIENTED_EDGE('',*,*,#13048,.T.);
#16577=ORIENTED_EDGE('',*,*,#13049,.T.);
#16578=ORIENTED_EDGE('',*,*,#13050,.T.);
#16579=ORIENTED_EDGE('',*,*,#13047,.F.);
#16580=ORIENTED_EDGE('',*,*,#13051,.T.);
#16581=ORIENTED_EDGE('',*,*,#13052,.F.);
#16582=ORIENTED_EDGE('',*,*,#13053,.F.);
#16583=ORIENTED_EDGE('',*,*,#13054,.F.);
#16584=ORIENTED_EDGE('',*,*,#13055,.F.);
#16585=ORIENTED_EDGE('',*,*,#13056,.F.);
#16586=ORIENTED_EDGE('',*,*,#13057,.F.);
#16587=ORIENTED_EDGE('',*,*,#13058,.F.);
#16588=ORIENTED_EDGE('',*,*,#13059,.F.);
#16589=ORIENTED_EDGE('',*,*,#13060,.F.);
#16590=ORIENTED_EDGE('',*,*,#13061,.F.);
#16591=ORIENTED_EDGE('',*,*,#13062,.F.);
#16592=ORIENTED_EDGE('',*,*,#13045,.F.);
#16593=ORIENTED_EDGE('',*,*,#13063,.F.);
#16594=ORIENTED_EDGE('',*,*,#13064,.F.);
#16595=ORIENTED_EDGE('',*,*,#13065,.F.);
#16596=ORIENTED_EDGE('',*,*,#13066,.F.);
#16597=ORIENTED_EDGE('',*,*,#13067,.F.);
#16598=ORIENTED_EDGE('',*,*,#13068,.F.);
#16599=ORIENTED_EDGE('',*,*,#13069,.F.);
#16600=ORIENTED_EDGE('',*,*,#13070,.F.);
#16601=ORIENTED_EDGE('',*,*,#13071,.F.);
#16602=ORIENTED_EDGE('',*,*,#13072,.F.);
#16603=ORIENTED_EDGE('',*,*,#13073,.F.);
#16604=ORIENTED_EDGE('',*,*,#13074,.F.);
#16605=ORIENTED_EDGE('',*,*,#13075,.F.);
#16606=ORIENTED_EDGE('',*,*,#13076,.F.);
#16607=ORIENTED_EDGE('',*,*,#13077,.F.);
#16608=ORIENTED_EDGE('',*,*,#13078,.F.);
#16609=ORIENTED_EDGE('',*,*,#13079,.F.);
#16610=ORIENTED_EDGE('',*,*,#13080,.F.);
#16611=ORIENTED_EDGE('',*,*,#13081,.F.);
#16612=ORIENTED_EDGE('',*,*,#13082,.F.);
#16613=ORIENTED_EDGE('',*,*,#13083,.F.);
#16614=ORIENTED_EDGE('',*,*,#13084,.F.);
#16615=ORIENTED_EDGE('',*,*,#13085,.F.);
#16616=ORIENTED_EDGE('',*,*,#13086,.F.);
#16617=ORIENTED_EDGE('',*,*,#13087,.F.);
#16618=ORIENTED_EDGE('',*,*,#13088,.F.);
#16619=ORIENTED_EDGE('',*,*,#13089,.F.);
#16620=ORIENTED_EDGE('',*,*,#13090,.F.);
#16621=ORIENTED_EDGE('',*,*,#13091,.F.);
#16622=ORIENTED_EDGE('',*,*,#13092,.T.);
#16623=ORIENTED_EDGE('',*,*,#13093,.T.);
#16624=ORIENTED_EDGE('',*,*,#13094,.F.);
#16625=ORIENTED_EDGE('',*,*,#13095,.T.);
#16626=ORIENTED_EDGE('',*,*,#13096,.F.);
#16627=ORIENTED_EDGE('',*,*,#13097,.F.);
#16628=ORIENTED_EDGE('',*,*,#13098,.F.);
#16629=ORIENTED_EDGE('',*,*,#13099,.F.);
#16630=ORIENTED_EDGE('',*,*,#13100,.F.);
#16631=ORIENTED_EDGE('',*,*,#13101,.F.);
#16632=ORIENTED_EDGE('',*,*,#13044,.F.);
#16633=ORIENTED_EDGE('',*,*,#13048,.F.);
#16634=ORIENTED_EDGE('',*,*,#13102,.T.);
#16635=ORIENTED_EDGE('',*,*,#13103,.F.);
#16636=ORIENTED_EDGE('',*,*,#13104,.F.);
#16637=ORIENTED_EDGE('',*,*,#13063,.T.);
#16638=ORIENTED_EDGE('',*,*,#13050,.F.);
#16639=ORIENTED_EDGE('',*,*,#13105,.F.);
#16640=ORIENTED_EDGE('',*,*,#13106,.F.);
#16641=ORIENTED_EDGE('',*,*,#13102,.F.);
#16642=ORIENTED_EDGE('',*,*,#13104,.T.);
#16643=ORIENTED_EDGE('',*,*,#13107,.F.);
#16644=ORIENTED_EDGE('',*,*,#13108,.T.);
#16645=ORIENTED_EDGE('',*,*,#13064,.T.);
#16646=ORIENTED_EDGE('',*,*,#13107,.T.);
#16647=ORIENTED_EDGE('',*,*,#13103,.T.);
#16648=ORIENTED_EDGE('',*,*,#13109,.T.);
#16649=ORIENTED_EDGE('',*,*,#13110,.T.);
#16650=ORIENTED_EDGE('',*,*,#13111,.T.);
#16651=ORIENTED_EDGE('',*,*,#13112,.T.);
#16652=ORIENTED_EDGE('',*,*,#13109,.F.);
#16653=ORIENTED_EDGE('',*,*,#13106,.T.);
#16654=ORIENTED_EDGE('',*,*,#13108,.F.);
#16655=ORIENTED_EDGE('',*,*,#13110,.F.);
#16656=ORIENTED_EDGE('',*,*,#13113,.T.);
#16657=ORIENTED_EDGE('',*,*,#13114,.F.);
#16658=ORIENTED_EDGE('',*,*,#13065,.T.);
#16659=ORIENTED_EDGE('',*,*,#13112,.F.);
#16660=ORIENTED_EDGE('',*,*,#13115,.F.);
#16661=ORIENTED_EDGE('',*,*,#13116,.F.);
#16662=ORIENTED_EDGE('',*,*,#13113,.F.);
#16663=ORIENTED_EDGE('',*,*,#13026,.T.);
#16664=ORIENTED_EDGE('',*,*,#13117,.T.);
#16665=ORIENTED_EDGE('',*,*,#13118,.T.);
#16666=ORIENTED_EDGE('',*,*,#13117,.F.);
#16667=ORIENTED_EDGE('',*,*,#13119,.F.);
#16668=ORIENTED_EDGE('',*,*,#13120,.T.);
#16669=ORIENTED_EDGE('',*,*,#13118,.F.);
#16670=ORIENTED_EDGE('',*,*,#13120,.F.);
#16671=ORIENTED_EDGE('',*,*,#13020,.T.);
#16672=ORIENTED_EDGE('',*,*,#13121,.T.);
#16673=ORIENTED_EDGE('',*,*,#13122,.T.);
#16674=ORIENTED_EDGE('',*,*,#13121,.F.);
#16675=ORIENTED_EDGE('',*,*,#13123,.F.);
#16676=ORIENTED_EDGE('',*,*,#13124,.T.);
#16677=ORIENTED_EDGE('',*,*,#13122,.F.);
#16678=ORIENTED_EDGE('',*,*,#13124,.F.);
#16679=ORIENTED_EDGE('',*,*,#13125,.T.);
#16680=ORIENTED_EDGE('',*,*,#13126,.T.);
#16681=ORIENTED_EDGE('',*,*,#13127,.T.);
#16682=ORIENTED_EDGE('',*,*,#13128,.T.);
#16683=ORIENTED_EDGE('',*,*,#13129,.F.);
#16684=ORIENTED_EDGE('',*,*,#13130,.T.);
#16685=ORIENTED_EDGE('',*,*,#13131,.T.);
#16686=ORIENTED_EDGE('',*,*,#13132,.F.);
#16687=ORIENTED_EDGE('',*,*,#13126,.F.);
#16688=ORIENTED_EDGE('',*,*,#13133,.F.);
#16689=ORIENTED_EDGE('',*,*,#13134,.F.);
#16690=ORIENTED_EDGE('',*,*,#13135,.F.);
#16691=ORIENTED_EDGE('',*,*,#13136,.T.);
#16692=ORIENTED_EDGE('',*,*,#13130,.F.);
#16693=ORIENTED_EDGE('',*,*,#13137,.T.);
#16694=ORIENTED_EDGE('',*,*,#13138,.T.);
#16695=ORIENTED_EDGE('',*,*,#13139,.T.);
#16696=ORIENTED_EDGE('',*,*,#13140,.T.);
#16697=ORIENTED_EDGE('',*,*,#13141,.F.);
#16698=ORIENTED_EDGE('',*,*,#13142,.T.);
#16699=ORIENTED_EDGE('',*,*,#13143,.F.);
#16700=ORIENTED_EDGE('',*,*,#13138,.F.);
#16701=ORIENTED_EDGE('',*,*,#13144,.F.);
#16702=ORIENTED_EDGE('',*,*,#13145,.T.);
#16703=ORIENTED_EDGE('',*,*,#13146,.F.);
#16704=ORIENTED_EDGE('',*,*,#13147,.F.);
#16705=ORIENTED_EDGE('',*,*,#13148,.F.);
#16706=ORIENTED_EDGE('',*,*,#13142,.F.);
#16707=ORIENTED_EDGE('',*,*,#13149,.T.);
#16708=ORIENTED_EDGE('',*,*,#13147,.T.);
#16709=ORIENTED_EDGE('',*,*,#13150,.T.);
#16710=ORIENTED_EDGE('',*,*,#13151,.T.);
#16711=ORIENTED_EDGE('',*,*,#13152,.T.);
#16712=ORIENTED_EDGE('',*,*,#13134,.T.);
#16713=ORIENTED_EDGE('',*,*,#13153,.T.);
#16714=ORIENTED_EDGE('',*,*,#13154,.T.);
#16715=ORIENTED_EDGE('',*,*,#13155,.T.);
#16716=ORIENTED_EDGE('',*,*,#13156,.T.);
#16717=ORIENTED_EDGE('',*,*,#13123,.T.);
#16718=ORIENTED_EDGE('',*,*,#13156,.F.);
#16719=ORIENTED_EDGE('',*,*,#13157,.F.);
#16720=ORIENTED_EDGE('',*,*,#13158,.F.);
#16721=ORIENTED_EDGE('',*,*,#13159,.F.);
#16722=ORIENTED_EDGE('',*,*,#13160,.F.);
#16723=ORIENTED_EDGE('',*,*,#13161,.F.);
#16724=ORIENTED_EDGE('',*,*,#13162,.F.);
#16725=ORIENTED_EDGE('',*,*,#13163,.F.);
#16726=ORIENTED_EDGE('',*,*,#13164,.F.);
#16727=ORIENTED_EDGE('',*,*,#13165,.F.);
#16728=ORIENTED_EDGE('',*,*,#13166,.F.);
#16729=ORIENTED_EDGE('',*,*,#13167,.F.);
#16730=ORIENTED_EDGE('',*,*,#13168,.F.);
#16731=ORIENTED_EDGE('',*,*,#13169,.F.);
#16732=ORIENTED_EDGE('',*,*,#13170,.F.);
#16733=ORIENTED_EDGE('',*,*,#13171,.F.);
#16734=ORIENTED_EDGE('',*,*,#13172,.T.);
#16735=ORIENTED_EDGE('',*,*,#13173,.T.);
#16736=ORIENTED_EDGE('',*,*,#13174,.F.);
#16737=ORIENTED_EDGE('',*,*,#13175,.F.);
#16738=ORIENTED_EDGE('',*,*,#13155,.F.);
#16739=ORIENTED_EDGE('',*,*,#13165,.T.);
#16740=ORIENTED_EDGE('',*,*,#13176,.T.);
#16741=ORIENTED_EDGE('',*,*,#13141,.T.);
#16742=ORIENTED_EDGE('',*,*,#13176,.F.);
#16743=ORIENTED_EDGE('',*,*,#13175,.T.);
#16744=ORIENTED_EDGE('',*,*,#13177,.T.);
#16745=ORIENTED_EDGE('',*,*,#13129,.T.);
#16746=ORIENTED_EDGE('',*,*,#13177,.F.);
#16747=ORIENTED_EDGE('',*,*,#13166,.T.);
#16748=ORIENTED_EDGE('',*,*,#13178,.T.);
#16749=ORIENTED_EDGE('',*,*,#13119,.T.);
#16750=ORIENTED_EDGE('',*,*,#13178,.F.);
#16751=ORIENTED_EDGE('',*,*,#13174,.T.);
#16752=ORIENTED_EDGE('',*,*,#13179,.T.);
#16753=ORIENTED_EDGE('',*,*,#13180,.T.);
#16754=ORIENTED_EDGE('',*,*,#13179,.F.);
#16755=ORIENTED_EDGE('',*,*,#13181,.F.);
#16756=ORIENTED_EDGE('',*,*,#13182,.T.);
#16757=ORIENTED_EDGE('',*,*,#13180,.F.);
#16758=ORIENTED_EDGE('',*,*,#13182,.F.);
#16759=ORIENTED_EDGE('',*,*,#13167,.T.);
#16760=ORIENTED_EDGE('',*,*,#13183,.T.);
#16761=ORIENTED_EDGE('',*,*,#13184,.T.);
#16762=ORIENTED_EDGE('',*,*,#13183,.F.);
#16763=ORIENTED_EDGE('',*,*,#13185,.F.);
#16764=ORIENTED_EDGE('',*,*,#13186,.T.);
#16765=ORIENTED_EDGE('',*,*,#13184,.F.);
#16766=ORIENTED_EDGE('',*,*,#13186,.F.);
#16767=ORIENTED_EDGE('',*,*,#13187,.T.);
#16768=ORIENTED_EDGE('',*,*,#13188,.F.);
#16769=ORIENTED_EDGE('',*,*,#13189,.T.);
#16770=ORIENTED_EDGE('',*,*,#13080,.T.);
#16771=ORIENTED_EDGE('',*,*,#13188,.T.);
#16772=ORIENTED_EDGE('',*,*,#13190,.T.);
#16773=ORIENTED_EDGE('',*,*,#13191,.T.);
#16774=ORIENTED_EDGE('',*,*,#13192,.T.);
#16775=ORIENTED_EDGE('',*,*,#13193,.T.);
#16776=ORIENTED_EDGE('',*,*,#13194,.T.);
#16777=ORIENTED_EDGE('',*,*,#13191,.F.);
#16778=ORIENTED_EDGE('',*,*,#13195,.T.);
#16779=ORIENTED_EDGE('',*,*,#13189,.F.);
#16780=ORIENTED_EDGE('',*,*,#13192,.F.);
#16781=ORIENTED_EDGE('',*,*,#13196,.T.);
#16782=ORIENTED_EDGE('',*,*,#13197,.F.);
#16783=ORIENTED_EDGE('',*,*,#13198,.F.);
#16784=ORIENTED_EDGE('',*,*,#13081,.T.);
#16785=ORIENTED_EDGE('',*,*,#13194,.F.);
#16786=ORIENTED_EDGE('',*,*,#13199,.F.);
#16787=ORIENTED_EDGE('',*,*,#13200,.F.);
#16788=ORIENTED_EDGE('',*,*,#13196,.F.);
#16789=ORIENTED_EDGE('',*,*,#13198,.T.);
#16790=ORIENTED_EDGE('',*,*,#13201,.F.);
#16791=ORIENTED_EDGE('',*,*,#13202,.T.);
#16792=ORIENTED_EDGE('',*,*,#13082,.T.);
#16793=ORIENTED_EDGE('',*,*,#13201,.T.);
#16794=ORIENTED_EDGE('',*,*,#13197,.T.);
#16795=ORIENTED_EDGE('',*,*,#13203,.T.);
#16796=ORIENTED_EDGE('',*,*,#13204,.T.);
#16797=ORIENTED_EDGE('',*,*,#13205,.T.);
#16798=ORIENTED_EDGE('',*,*,#13206,.T.);
#16799=ORIENTED_EDGE('',*,*,#13203,.F.);
#16800=ORIENTED_EDGE('',*,*,#13200,.T.);
#16801=ORIENTED_EDGE('',*,*,#13202,.F.);
#16802=ORIENTED_EDGE('',*,*,#13204,.F.);
#16803=ORIENTED_EDGE('',*,*,#13207,.T.);
#16804=ORIENTED_EDGE('',*,*,#13208,.F.);
#16805=ORIENTED_EDGE('',*,*,#13083,.T.);
#16806=ORIENTED_EDGE('',*,*,#13206,.F.);
#16807=ORIENTED_EDGE('',*,*,#13209,.F.);
#16808=ORIENTED_EDGE('',*,*,#13210,.F.);
#16809=ORIENTED_EDGE('',*,*,#13207,.F.);
#16810=ORIENTED_EDGE('',*,*,#13101,.T.);
#16811=ORIENTED_EDGE('',*,*,#13211,.T.);
#16812=ORIENTED_EDGE('',*,*,#13185,.T.);
#16813=ORIENTED_EDGE('',*,*,#13211,.F.);
#16814=ORIENTED_EDGE('',*,*,#13062,.T.);
#16815=ORIENTED_EDGE('',*,*,#13212,.T.);
#16816=ORIENTED_EDGE('',*,*,#13181,.T.);
#16817=ORIENTED_EDGE('',*,*,#13212,.F.);
#16818=ORIENTED_EDGE('',*,*,#13213,.T.);
#16819=ORIENTED_EDGE('',*,*,#13214,.T.);
#16820=ORIENTED_EDGE('',*,*,#13215,.T.);
#16821=ORIENTED_EDGE('',*,*,#13216,.T.);
#16822=ORIENTED_EDGE('',*,*,#13217,.T.);
#16823=ORIENTED_EDGE('',*,*,#13218,.T.);
#16824=ORIENTED_EDGE('',*,*,#13215,.F.);
#16825=ORIENTED_EDGE('',*,*,#13219,.T.);
#16826=ORIENTED_EDGE('',*,*,#13220,.T.);
#16827=ORIENTED_EDGE('',*,*,#13068,.T.);
#16828=ORIENTED_EDGE('',*,*,#13217,.F.);
#16829=ORIENTED_EDGE('',*,*,#13221,.T.);
#16830=ORIENTED_EDGE('',*,*,#13222,.T.);
#16831=ORIENTED_EDGE('',*,*,#13223,.T.);
#16832=ORIENTED_EDGE('',*,*,#13220,.F.);
#16833=ORIENTED_EDGE('',*,*,#13224,.T.);
#16834=ORIENTED_EDGE('',*,*,#13225,.T.);
#16835=ORIENTED_EDGE('',*,*,#13226,.T.);
#16836=ORIENTED_EDGE('',*,*,#13222,.F.);
#16837=ORIENTED_EDGE('',*,*,#13227,.T.);
#16838=ORIENTED_EDGE('',*,*,#13227,.F.);
#16839=ORIENTED_EDGE('',*,*,#13224,.F.);
#16840=ORIENTED_EDGE('',*,*,#13221,.F.);
#16841=ORIENTED_EDGE('',*,*,#13219,.F.);
#16842=ORIENTED_EDGE('',*,*,#13214,.F.);
#16843=ORIENTED_EDGE('',*,*,#13228,.F.);
#16844=ORIENTED_EDGE('',*,*,#13229,.T.);
#16845=ORIENTED_EDGE('',*,*,#13230,.T.);
#16846=ORIENTED_EDGE('',*,*,#13231,.T.);
#16847=ORIENTED_EDGE('',*,*,#13232,.T.);
#16848=ORIENTED_EDGE('',*,*,#13230,.F.);
#16849=ORIENTED_EDGE('',*,*,#13233,.F.);
#16850=ORIENTED_EDGE('',*,*,#13234,.F.);
#16851=ORIENTED_EDGE('',*,*,#13235,.F.);
#16852=ORIENTED_EDGE('',*,*,#13099,.T.);
#16853=ORIENTED_EDGE('',*,*,#13236,.T.);
#16854=ORIENTED_EDGE('',*,*,#13237,.T.);
#16855=ORIENTED_EDGE('',*,*,#13238,.F.);
#16856=ORIENTED_EDGE('',*,*,#13098,.T.);
#16857=ORIENTED_EDGE('',*,*,#13239,.T.);
#16858=ORIENTED_EDGE('',*,*,#13240,.T.);
#16859=ORIENTED_EDGE('',*,*,#13236,.F.);
#16860=ORIENTED_EDGE('',*,*,#13241,.T.);
#16861=ORIENTED_EDGE('',*,*,#13242,.T.);
#16862=ORIENTED_EDGE('',*,*,#13243,.T.);
#16863=ORIENTED_EDGE('',*,*,#13096,.T.);
#16864=ORIENTED_EDGE('',*,*,#13097,.T.);
#16865=ORIENTED_EDGE('',*,*,#13243,.F.);
#16866=ORIENTED_EDGE('',*,*,#13244,.T.);
#16867=ORIENTED_EDGE('',*,*,#13239,.F.);
#16868=ORIENTED_EDGE('',*,*,#13245,.T.);
#16869=ORIENTED_EDGE('',*,*,#13241,.F.);
#16870=ORIENTED_EDGE('',*,*,#13100,.T.);
#16871=ORIENTED_EDGE('',*,*,#13238,.T.);
#16872=ORIENTED_EDGE('',*,*,#13240,.F.);
#16873=ORIENTED_EDGE('',*,*,#13246,.F.);
#16874=ORIENTED_EDGE('',*,*,#13247,.F.);
#16875=ORIENTED_EDGE('',*,*,#13248,.T.);
#16876=ORIENTED_EDGE('',*,*,#13244,.F.);
#16877=ORIENTED_EDGE('',*,*,#13249,.T.);
#16878=ORIENTED_EDGE('',*,*,#13250,.T.);
#16879=ORIENTED_EDGE('',*,*,#13246,.T.);
#16880=ORIENTED_EDGE('',*,*,#13242,.F.);
#16881=ORIENTED_EDGE('',*,*,#13251,.T.);
#16882=ORIENTED_EDGE('',*,*,#13252,.T.);
#16883=ORIENTED_EDGE('',*,*,#13249,.F.);
#16884=ORIENTED_EDGE('',*,*,#13089,.T.);
#16885=ORIENTED_EDGE('',*,*,#13253,.T.);
#16886=ORIENTED_EDGE('',*,*,#13254,.T.);
#16887=ORIENTED_EDGE('',*,*,#13255,.F.);
#16888=ORIENTED_EDGE('',*,*,#13088,.T.);
#16889=ORIENTED_EDGE('',*,*,#13256,.T.);
#16890=ORIENTED_EDGE('',*,*,#13257,.T.);
#16891=ORIENTED_EDGE('',*,*,#13253,.F.);
#16892=ORIENTED_EDGE('',*,*,#13258,.T.);
#16893=ORIENTED_EDGE('',*,*,#13259,.T.);
#16894=ORIENTED_EDGE('',*,*,#13260,.T.);
#16895=ORIENTED_EDGE('',*,*,#13086,.T.);
#16896=ORIENTED_EDGE('',*,*,#13087,.T.);
#16897=ORIENTED_EDGE('',*,*,#13260,.F.);
#16898=ORIENTED_EDGE('',*,*,#13261,.T.);
#16899=ORIENTED_EDGE('',*,*,#13256,.F.);
#16900=ORIENTED_EDGE('',*,*,#13262,.T.);
#16901=ORIENTED_EDGE('',*,*,#13258,.F.);
#16902=ORIENTED_EDGE('',*,*,#13090,.T.);
#16903=ORIENTED_EDGE('',*,*,#13255,.T.);
#16904=ORIENTED_EDGE('',*,*,#13257,.F.);
#16905=ORIENTED_EDGE('',*,*,#13263,.F.);
#16906=ORIENTED_EDGE('',*,*,#13264,.F.);
#16907=ORIENTED_EDGE('',*,*,#13265,.T.);
#16908=ORIENTED_EDGE('',*,*,#13261,.F.);
#16909=ORIENTED_EDGE('',*,*,#13266,.T.);
#16910=ORIENTED_EDGE('',*,*,#13267,.T.);
#16911=ORIENTED_EDGE('',*,*,#13263,.T.);
#16912=ORIENTED_EDGE('',*,*,#13259,.F.);
#16913=ORIENTED_EDGE('',*,*,#13268,.T.);
#16914=ORIENTED_EDGE('',*,*,#13269,.T.);
#16915=ORIENTED_EDGE('',*,*,#13266,.F.);
#16916=ORIENTED_EDGE('',*,*,#13270,.T.);
#16917=ORIENTED_EDGE('',*,*,#13234,.T.);
#16918=ORIENTED_EDGE('',*,*,#13271,.T.);
#16919=ORIENTED_EDGE('',*,*,#13061,.T.);
#16920=ORIENTED_EDGE('',*,*,#13114,.T.);
#16921=ORIENTED_EDGE('',*,*,#13272,.T.);
#16922=ORIENTED_EDGE('',*,*,#13273,.T.);
#16923=ORIENTED_EDGE('',*,*,#13066,.T.);
#16924=ORIENTED_EDGE('',*,*,#13272,.F.);
#16925=ORIENTED_EDGE('',*,*,#13116,.T.);
#16926=ORIENTED_EDGE('',*,*,#13274,.F.);
#16927=ORIENTED_EDGE('',*,*,#13275,.T.);
#16928=ORIENTED_EDGE('',*,*,#13276,.T.);
#16929=ORIENTED_EDGE('',*,*,#13277,.T.);
#16930=ORIENTED_EDGE('',*,*,#13278,.T.);
#16931=ORIENTED_EDGE('',*,*,#13077,.T.);
#16932=ORIENTED_EDGE('',*,*,#13277,.F.);
#16933=ORIENTED_EDGE('',*,*,#13279,.F.);
#16934=ORIENTED_EDGE('',*,*,#13280,.F.);
#16935=ORIENTED_EDGE('',*,*,#13281,.T.);
#16936=ORIENTED_EDGE('',*,*,#13282,.T.);
#16937=ORIENTED_EDGE('',*,*,#13283,.T.);
#16938=ORIENTED_EDGE('',*,*,#13072,.T.);
#16939=ORIENTED_EDGE('',*,*,#13284,.T.);
#16940=ORIENTED_EDGE('',*,*,#13071,.T.);
#16941=ORIENTED_EDGE('',*,*,#13285,.T.);
#16942=ORIENTED_EDGE('',*,*,#13286,.T.);
#16943=ORIENTED_EDGE('',*,*,#13284,.F.);
#16944=ORIENTED_EDGE('',*,*,#13070,.T.);
#16945=ORIENTED_EDGE('',*,*,#13287,.T.);
#16946=ORIENTED_EDGE('',*,*,#13288,.T.);
#16947=ORIENTED_EDGE('',*,*,#13285,.F.);
#16948=ORIENTED_EDGE('',*,*,#13289,.T.);
#16949=ORIENTED_EDGE('',*,*,#13073,.T.);
#16950=ORIENTED_EDGE('',*,*,#13283,.F.);
#16951=ORIENTED_EDGE('',*,*,#13290,.T.);
#16952=ORIENTED_EDGE('',*,*,#13291,.T.);
#16953=ORIENTED_EDGE('',*,*,#13074,.T.);
#16954=ORIENTED_EDGE('',*,*,#13289,.F.);
#16955=ORIENTED_EDGE('',*,*,#13292,.T.);
#16956=ORIENTED_EDGE('',*,*,#13293,.T.);
#16957=ORIENTED_EDGE('',*,*,#13075,.T.);
#16958=ORIENTED_EDGE('',*,*,#13291,.F.);
#16959=ORIENTED_EDGE('',*,*,#13294,.T.);
#16960=ORIENTED_EDGE('',*,*,#13076,.T.);
#16961=ORIENTED_EDGE('',*,*,#13293,.F.);
#16962=ORIENTED_EDGE('',*,*,#13295,.T.);
#16963=ORIENTED_EDGE('',*,*,#13276,.F.);
#16964=ORIENTED_EDGE('',*,*,#13295,.F.);
#16965=ORIENTED_EDGE('',*,*,#13296,.T.);
#16966=ORIENTED_EDGE('',*,*,#13297,.T.);
#16967=ORIENTED_EDGE('',*,*,#13279,.T.);
#16968=ORIENTED_EDGE('',*,*,#13294,.F.);
#16969=ORIENTED_EDGE('',*,*,#13298,.T.);
#16970=ORIENTED_EDGE('',*,*,#13299,.T.);
#16971=ORIENTED_EDGE('',*,*,#13296,.F.);
#16972=ORIENTED_EDGE('',*,*,#13292,.F.);
#16973=ORIENTED_EDGE('',*,*,#13300,.T.);
#16974=ORIENTED_EDGE('',*,*,#13301,.T.);
#16975=ORIENTED_EDGE('',*,*,#13298,.F.);
#16976=ORIENTED_EDGE('',*,*,#13290,.F.);
#16977=ORIENTED_EDGE('',*,*,#13302,.T.);
#16978=ORIENTED_EDGE('',*,*,#13303,.T.);
#16979=ORIENTED_EDGE('',*,*,#13300,.F.);
#16980=ORIENTED_EDGE('',*,*,#13282,.F.);
#16981=ORIENTED_EDGE('',*,*,#13304,.T.);
#16982=ORIENTED_EDGE('',*,*,#13305,.T.);
#16983=ORIENTED_EDGE('',*,*,#13302,.F.);
#16984=ORIENTED_EDGE('',*,*,#13286,.F.);
#16985=ORIENTED_EDGE('',*,*,#13306,.F.);
#16986=ORIENTED_EDGE('',*,*,#13307,.F.);
#16987=ORIENTED_EDGE('',*,*,#13304,.F.);
#16988=ORIENTED_EDGE('',*,*,#13288,.F.);
#16989=ORIENTED_EDGE('',*,*,#13308,.T.);
#16990=ORIENTED_EDGE('',*,*,#13309,.F.);
#16991=ORIENTED_EDGE('',*,*,#13306,.T.);
#16992=ORIENTED_EDGE('',*,*,#13310,.T.);
#16993=ORIENTED_EDGE('',*,*,#13311,.T.);
#16994=ORIENTED_EDGE('',*,*,#13312,.T.);
#16995=ORIENTED_EDGE('',*,*,#13054,.T.);
#16996=ORIENTED_EDGE('',*,*,#13313,.T.);
#16997=ORIENTED_EDGE('',*,*,#13055,.T.);
#16998=ORIENTED_EDGE('',*,*,#13312,.F.);
#16999=ORIENTED_EDGE('',*,*,#13314,.T.);
#17000=ORIENTED_EDGE('',*,*,#13315,.T.);
#17001=ORIENTED_EDGE('',*,*,#13056,.T.);
#17002=ORIENTED_EDGE('',*,*,#13313,.F.);
#17003=ORIENTED_EDGE('',*,*,#13316,.T.);
#17004=ORIENTED_EDGE('',*,*,#13317,.T.);
#17005=ORIENTED_EDGE('',*,*,#13057,.T.);
#17006=ORIENTED_EDGE('',*,*,#13315,.F.);
#17007=ORIENTED_EDGE('',*,*,#13318,.T.);
#17008=ORIENTED_EDGE('',*,*,#13319,.T.);
#17009=ORIENTED_EDGE('',*,*,#13058,.T.);
#17010=ORIENTED_EDGE('',*,*,#13317,.F.);
#17011=ORIENTED_EDGE('',*,*,#13320,.T.);
#17012=ORIENTED_EDGE('',*,*,#13321,.T.);
#17013=ORIENTED_EDGE('',*,*,#13059,.T.);
#17014=ORIENTED_EDGE('',*,*,#13319,.F.);
#17015=ORIENTED_EDGE('',*,*,#13322,.T.);
#17016=ORIENTED_EDGE('',*,*,#13060,.T.);
#17017=ORIENTED_EDGE('',*,*,#13321,.F.);
#17018=ORIENTED_EDGE('',*,*,#13323,.T.);
#17019=ORIENTED_EDGE('',*,*,#13270,.F.);
#17020=ORIENTED_EDGE('',*,*,#13324,.T.);
#17021=ORIENTED_EDGE('',*,*,#13325,.T.);
#17022=ORIENTED_EDGE('',*,*,#13310,.F.);
#17023=ORIENTED_EDGE('',*,*,#13053,.T.);
#17024=ORIENTED_EDGE('',*,*,#13326,.T.);
#17025=ORIENTED_EDGE('',*,*,#13324,.F.);
#17026=ORIENTED_EDGE('',*,*,#13052,.T.);
#17027=ORIENTED_EDGE('',*,*,#13271,.F.);
#17028=ORIENTED_EDGE('',*,*,#13318,.F.);
#17029=ORIENTED_EDGE('',*,*,#13327,.T.);
#17030=ORIENTED_EDGE('',*,*,#13328,.F.);
#17031=ORIENTED_EDGE('',*,*,#13329,.F.);
#17032=ORIENTED_EDGE('',*,*,#13316,.F.);
#17033=ORIENTED_EDGE('',*,*,#13330,.T.);
#17034=ORIENTED_EDGE('',*,*,#13331,.F.);
#17035=ORIENTED_EDGE('',*,*,#13327,.F.);
#17036=ORIENTED_EDGE('',*,*,#13314,.F.);
#17037=ORIENTED_EDGE('',*,*,#13332,.T.);
#17038=ORIENTED_EDGE('',*,*,#13333,.F.);
#17039=ORIENTED_EDGE('',*,*,#13330,.F.);
#17040=ORIENTED_EDGE('',*,*,#13311,.F.);
#17041=ORIENTED_EDGE('',*,*,#13334,.T.);
#17042=ORIENTED_EDGE('',*,*,#13335,.F.);
#17043=ORIENTED_EDGE('',*,*,#13332,.F.);
#17044=ORIENTED_EDGE('',*,*,#13325,.F.);
#17045=ORIENTED_EDGE('',*,*,#13336,.T.);
#17046=ORIENTED_EDGE('',*,*,#13337,.F.);
#17047=ORIENTED_EDGE('',*,*,#13334,.F.);
#17048=ORIENTED_EDGE('',*,*,#13223,.F.);
#17049=ORIENTED_EDGE('',*,*,#13338,.T.);
#17050=ORIENTED_EDGE('',*,*,#13287,.F.);
#17051=ORIENTED_EDGE('',*,*,#13069,.T.);
#17052=ORIENTED_EDGE('',*,*,#13226,.F.);
#17053=ORIENTED_EDGE('',*,*,#13339,.F.);
#17054=ORIENTED_EDGE('',*,*,#13308,.F.);
#17055=ORIENTED_EDGE('',*,*,#13338,.F.);
#17056=ORIENTED_EDGE('',*,*,#13218,.F.);
#17057=ORIENTED_EDGE('',*,*,#13067,.T.);
#17058=ORIENTED_EDGE('',*,*,#13273,.F.);
#17059=ORIENTED_EDGE('',*,*,#13340,.T.);
#17060=ORIENTED_EDGE('',*,*,#13216,.F.);
#17061=ORIENTED_EDGE('',*,*,#13340,.F.);
#17062=ORIENTED_EDGE('',*,*,#13275,.F.);
#17063=ORIENTED_EDGE('',*,*,#13341,.F.);
#17064=ORIENTED_EDGE('',*,*,#13342,.T.);
#17065=ORIENTED_EDGE('',*,*,#13343,.T.);
#17066=ORIENTED_EDGE('',*,*,#13084,.T.);
#17067=ORIENTED_EDGE('',*,*,#13208,.T.);
#17068=ORIENTED_EDGE('',*,*,#13187,.F.);
#17069=ORIENTED_EDGE('',*,*,#13079,.T.);
#17070=ORIENTED_EDGE('',*,*,#13344,.T.);
#17071=ORIENTED_EDGE('',*,*,#13345,.T.);
#17072=ORIENTED_EDGE('',*,*,#13190,.F.);
#17073=ORIENTED_EDGE('',*,*,#13078,.T.);
#17074=ORIENTED_EDGE('',*,*,#13278,.F.);
#17075=ORIENTED_EDGE('',*,*,#13346,.T.);
#17076=ORIENTED_EDGE('',*,*,#13344,.F.);
#17077=ORIENTED_EDGE('',*,*,#13342,.F.);
#17078=ORIENTED_EDGE('',*,*,#13210,.T.);
#17079=ORIENTED_EDGE('',*,*,#13347,.F.);
#17080=ORIENTED_EDGE('',*,*,#13348,.T.);
#17081=ORIENTED_EDGE('',*,*,#13195,.F.);
#17082=ORIENTED_EDGE('',*,*,#13345,.F.);
#17083=ORIENTED_EDGE('',*,*,#13349,.F.);
#17084=ORIENTED_EDGE('',*,*,#13350,.F.);
#17085=ORIENTED_EDGE('',*,*,#13346,.F.);
#17086=ORIENTED_EDGE('',*,*,#13281,.F.);
#17087=ORIENTED_EDGE('',*,*,#13351,.F.);
#17088=ORIENTED_EDGE('',*,*,#13349,.T.);
#17089=ORIENTED_EDGE('',*,*,#13352,.T.);
#17090=ORIENTED_EDGE('',*,*,#13328,.T.);
#17091=ORIENTED_EDGE('',*,*,#13353,.T.);
#17092=ORIENTED_EDGE('',*,*,#13157,.T.);
#17093=ORIENTED_EDGE('',*,*,#13354,.T.);
#17094=ORIENTED_EDGE('',*,*,#13158,.T.);
#17095=ORIENTED_EDGE('',*,*,#13353,.F.);
#17096=ORIENTED_EDGE('',*,*,#13331,.T.);
#17097=ORIENTED_EDGE('',*,*,#13355,.T.);
#17098=ORIENTED_EDGE('',*,*,#13159,.T.);
#17099=ORIENTED_EDGE('',*,*,#13354,.F.);
#17100=ORIENTED_EDGE('',*,*,#13333,.T.);
#17101=ORIENTED_EDGE('',*,*,#13356,.T.);
#17102=ORIENTED_EDGE('',*,*,#13160,.T.);
#17103=ORIENTED_EDGE('',*,*,#13355,.F.);
#17104=ORIENTED_EDGE('',*,*,#13335,.T.);
#17105=ORIENTED_EDGE('',*,*,#13357,.T.);
#17106=ORIENTED_EDGE('',*,*,#13161,.T.);
#17107=ORIENTED_EDGE('',*,*,#13356,.F.);
#17108=ORIENTED_EDGE('',*,*,#13337,.T.);
#17109=ORIENTED_EDGE('',*,*,#13358,.T.);
#17110=ORIENTED_EDGE('',*,*,#13162,.T.);
#17111=ORIENTED_EDGE('',*,*,#13357,.F.);
#17112=ORIENTED_EDGE('',*,*,#13359,.T.);
#17113=ORIENTED_EDGE('',*,*,#13360,.T.);
#17114=ORIENTED_EDGE('',*,*,#13163,.T.);
#17115=ORIENTED_EDGE('',*,*,#13358,.F.);
#17116=ORIENTED_EDGE('',*,*,#13361,.T.);
#17117=ORIENTED_EDGE('',*,*,#13352,.F.);
#17118=ORIENTED_EDGE('',*,*,#13164,.T.);
#17119=ORIENTED_EDGE('',*,*,#13360,.F.);
#17120=ORIENTED_EDGE('',*,*,#13362,.T.);
#17121=ORIENTED_EDGE('',*,*,#13363,.T.);
#17122=ORIENTED_EDGE('',*,*,#13364,.T.);
#17123=ORIENTED_EDGE('',*,*,#13365,.T.);
#17124=ORIENTED_EDGE('',*,*,#13364,.F.);
#17125=ORIENTED_EDGE('',*,*,#13366,.F.);
#17126=ORIENTED_EDGE('',*,*,#13154,.F.);
#17127=ORIENTED_EDGE('',*,*,#13367,.F.);
#17128=ORIENTED_EDGE('',*,*,#13095,.F.);
#17129=ORIENTED_EDGE('',*,*,#13368,.F.);
#17130=ORIENTED_EDGE('',*,*,#13151,.F.);
#17131=ORIENTED_EDGE('',*,*,#13369,.F.);
#17132=ORIENTED_EDGE('',*,*,#13140,.F.);
#17133=ORIENTED_EDGE('',*,*,#13370,.F.);
#17134=ORIENTED_EDGE('',*,*,#13093,.F.);
#17135=ORIENTED_EDGE('',*,*,#13371,.T.);
#17136=ORIENTED_EDGE('',*,*,#13363,.F.);
#17137=ORIENTED_EDGE('',*,*,#13371,.F.);
#17138=ORIENTED_EDGE('',*,*,#13092,.F.);
#17139=ORIENTED_EDGE('',*,*,#13372,.F.);
#17140=ORIENTED_EDGE('',*,*,#13128,.F.);
#17141=ORIENTED_EDGE('',*,*,#13365,.F.);
#17142=ORIENTED_EDGE('',*,*,#13373,.T.);
#17143=ORIENTED_EDGE('',*,*,#13042,.F.);
#17144=ORIENTED_EDGE('',*,*,#13085,.T.);
#17145=ORIENTED_EDGE('',*,*,#13343,.F.);
#17146=ORIENTED_EDGE('',*,*,#13374,.T.);
#17147=ORIENTED_EDGE('',*,*,#13046,.F.);
#17148=ORIENTED_EDGE('',*,*,#13051,.F.);
#17149=ORIENTED_EDGE('',*,*,#13374,.F.);
#17150=ORIENTED_EDGE('',*,*,#13348,.F.);
#17151=ORIENTED_EDGE('',*,*,#13375,.F.);
#17152=ORIENTED_EDGE('',*,*,#13367,.T.);
#17153=ORIENTED_EDGE('',*,*,#13153,.F.);
#17154=ORIENTED_EDGE('',*,*,#13133,.T.);
#17155=ORIENTED_EDGE('',*,*,#13125,.F.);
#17156=ORIENTED_EDGE('',*,*,#13372,.T.);
#17157=ORIENTED_EDGE('',*,*,#13091,.T.);
#17158=ORIENTED_EDGE('',*,*,#13132,.T.);
#17159=ORIENTED_EDGE('',*,*,#13376,.T.);
#17160=ORIENTED_EDGE('',*,*,#13135,.T.);
#17161=ORIENTED_EDGE('',*,*,#13152,.F.);
#17162=ORIENTED_EDGE('',*,*,#13366,.T.);
#17163=ORIENTED_EDGE('',*,*,#13127,.F.);
#17164=ORIENTED_EDGE('',*,*,#13376,.F.);
#17165=ORIENTED_EDGE('',*,*,#13131,.F.);
#17166=ORIENTED_EDGE('',*,*,#13136,.F.);
#17167=ORIENTED_EDGE('',*,*,#13370,.T.);
#17168=ORIENTED_EDGE('',*,*,#13139,.F.);
#17169=ORIENTED_EDGE('',*,*,#13143,.T.);
#17170=ORIENTED_EDGE('',*,*,#13148,.T.);
#17171=ORIENTED_EDGE('',*,*,#13149,.F.);
#17172=ORIENTED_EDGE('',*,*,#13368,.T.);
#17173=ORIENTED_EDGE('',*,*,#13094,.T.);
#17174=ORIENTED_EDGE('',*,*,#13146,.T.);
#17175=ORIENTED_EDGE('',*,*,#13377,.T.);
#17176=ORIENTED_EDGE('',*,*,#13144,.T.);
#17177=ORIENTED_EDGE('',*,*,#13137,.F.);
#17178=ORIENTED_EDGE('',*,*,#13369,.T.);
#17179=ORIENTED_EDGE('',*,*,#13150,.F.);
#17180=ORIENTED_EDGE('',*,*,#13377,.F.);
#17181=ORIENTED_EDGE('',*,*,#13145,.F.);
#17182=ORIENTED_EDGE('',*,*,#13378,.T.);
#17183=ORIENTED_EDGE('',*,*,#13379,.T.);
#17184=ORIENTED_EDGE('',*,*,#13380,.T.);
#17185=ORIENTED_EDGE('',*,*,#13168,.T.);
#17186=ORIENTED_EDGE('',*,*,#13381,.T.);
#17187=ORIENTED_EDGE('',*,*,#13169,.T.);
#17188=ORIENTED_EDGE('',*,*,#13380,.F.);
#17189=ORIENTED_EDGE('',*,*,#13382,.T.);
#17190=ORIENTED_EDGE('',*,*,#13383,.T.);
#17191=ORIENTED_EDGE('',*,*,#13170,.T.);
#17192=ORIENTED_EDGE('',*,*,#13381,.F.);
#17193=ORIENTED_EDGE('',*,*,#13384,.T.);
#17194=ORIENTED_EDGE('',*,*,#13378,.F.);
#17195=ORIENTED_EDGE('',*,*,#13171,.T.);
#17196=ORIENTED_EDGE('',*,*,#13383,.F.);
#17197=ORIENTED_EDGE('',*,*,#13385,.T.);
#17198=ORIENTED_EDGE('',*,*,#13382,.F.);
#17199=ORIENTED_EDGE('',*,*,#13386,.T.);
#17200=ORIENTED_EDGE('',*,*,#13387,.T.);
#17201=ORIENTED_EDGE('',*,*,#13388,.F.);
#17202=ORIENTED_EDGE('',*,*,#13379,.F.);
#17203=ORIENTED_EDGE('',*,*,#13389,.T.);
#17204=ORIENTED_EDGE('',*,*,#13390,.T.);
#17205=ORIENTED_EDGE('',*,*,#13386,.F.);
#17206=ORIENTED_EDGE('',*,*,#13391,.T.);
#17207=ORIENTED_EDGE('',*,*,#13392,.T.);
#17208=ORIENTED_EDGE('',*,*,#13393,.T.);
#17209=ORIENTED_EDGE('',*,*,#13038,.T.);
#17210=ORIENTED_EDGE('',*,*,#13394,.T.);
#17211=ORIENTED_EDGE('',*,*,#13039,.T.);
#17212=ORIENTED_EDGE('',*,*,#13393,.F.);
#17213=ORIENTED_EDGE('',*,*,#13395,.T.);
#17214=ORIENTED_EDGE('',*,*,#13396,.T.);
#17215=ORIENTED_EDGE('',*,*,#13040,.T.);
#17216=ORIENTED_EDGE('',*,*,#13394,.F.);
#17217=ORIENTED_EDGE('',*,*,#13397,.T.);
#17218=ORIENTED_EDGE('',*,*,#13391,.F.);
#17219=ORIENTED_EDGE('',*,*,#13041,.T.);
#17220=ORIENTED_EDGE('',*,*,#13396,.F.);
#17221=ORIENTED_EDGE('',*,*,#13398,.T.);
#17222=ORIENTED_EDGE('',*,*,#13395,.F.);
#17223=ORIENTED_EDGE('',*,*,#13399,.T.);
#17224=ORIENTED_EDGE('',*,*,#13400,.T.);
#17225=ORIENTED_EDGE('',*,*,#13401,.F.);
#17226=ORIENTED_EDGE('',*,*,#13392,.F.);
#17227=ORIENTED_EDGE('',*,*,#13402,.T.);
#17228=ORIENTED_EDGE('',*,*,#13403,.T.);
#17229=ORIENTED_EDGE('',*,*,#13399,.F.);
#17230=ORIENTED_EDGE('',*,*,#13398,.F.);
#17231=ORIENTED_EDGE('',*,*,#13404,.T.);
#17232=ORIENTED_EDGE('',*,*,#13405,.T.);
#17233=ORIENTED_EDGE('',*,*,#13402,.F.);
#17234=ORIENTED_EDGE('',*,*,#13397,.F.);
#17235=ORIENTED_EDGE('',*,*,#13401,.T.);
#17236=ORIENTED_EDGE('',*,*,#13406,.T.);
#17237=ORIENTED_EDGE('',*,*,#13404,.F.);
#17238=ORIENTED_EDGE('',*,*,#13385,.F.);
#17239=ORIENTED_EDGE('',*,*,#13407,.T.);
#17240=ORIENTED_EDGE('',*,*,#13408,.T.);
#17241=ORIENTED_EDGE('',*,*,#13389,.F.);
#17242=ORIENTED_EDGE('',*,*,#13384,.F.);
#17243=ORIENTED_EDGE('',*,*,#13388,.T.);
#17244=ORIENTED_EDGE('',*,*,#13409,.T.);
#17245=ORIENTED_EDGE('',*,*,#13407,.F.);
#17246=ORIENTED_EDGE('',*,*,#13387,.F.);
#17247=ORIENTED_EDGE('',*,*,#13390,.F.);
#17248=ORIENTED_EDGE('',*,*,#13408,.F.);
#17249=ORIENTED_EDGE('',*,*,#13409,.F.);
#17250=ORIENTED_EDGE('',*,*,#13400,.F.);
#17251=ORIENTED_EDGE('',*,*,#13403,.F.);
#17252=ORIENTED_EDGE('',*,*,#13405,.F.);
#17253=ORIENTED_EDGE('',*,*,#13406,.F.);
#17254=ORIENTED_EDGE('',*,*,#13172,.F.);
#17255=ORIENTED_EDGE('',*,*,#13410,.T.);
#17256=ORIENTED_EDGE('',*,*,#13411,.T.);
#17257=ORIENTED_EDGE('',*,*,#13410,.F.);
#17258=ORIENTED_EDGE('',*,*,#13411,.F.);
#17259=ORIENTED_EDGE('',*,*,#13173,.F.);
#17260=ORIENTED_EDGE('',*,*,#13412,.T.);
#17261=ORIENTED_EDGE('',*,*,#13413,.T.);
#17262=ORIENTED_EDGE('',*,*,#13412,.F.);
#17263=ORIENTED_EDGE('',*,*,#13413,.F.);
#17264=ORIENTED_EDGE('',*,*,#13414,.T.);
#17265=ORIENTED_EDGE('',*,*,#13415,.F.);
#17266=ORIENTED_EDGE('',*,*,#13414,.F.);
#17267=ORIENTED_EDGE('',*,*,#13416,.T.);
#17268=ORIENTED_EDGE('',*,*,#13417,.T.);
#17269=ORIENTED_EDGE('',*,*,#13416,.F.);
#17270=ORIENTED_EDGE('',*,*,#13417,.F.);
#17271=ORIENTED_EDGE('',*,*,#13418,.F.);
#17272=ORIENTED_EDGE('',*,*,#13418,.T.);
#17273=ORIENTED_EDGE('',*,*,#13419,.T.);
#17274=ORIENTED_EDGE('',*,*,#13035,.T.);
#17275=ORIENTED_EDGE('',*,*,#13419,.F.);
#17276=ORIENTED_EDGE('',*,*,#13373,.F.);
#17277=ORIENTED_EDGE('',*,*,#13420,.T.);
#17278=ORIENTED_EDGE('',*,*,#13415,.T.);
#17279=ORIENTED_EDGE('',*,*,#13420,.F.);
#17280=ORIENTED_EDGE('',*,*,#13115,.T.);
#17281=ORIENTED_EDGE('',*,*,#13111,.F.);
#17282=ORIENTED_EDGE('',*,*,#13105,.T.);
#17283=ORIENTED_EDGE('',*,*,#13049,.F.);
#17284=ORIENTED_EDGE('',*,*,#13375,.T.);
#17285=ORIENTED_EDGE('',*,*,#13347,.T.);
#17286=ORIENTED_EDGE('',*,*,#13209,.T.);
#17287=ORIENTED_EDGE('',*,*,#13205,.F.);
#17288=ORIENTED_EDGE('',*,*,#13199,.T.);
#17289=ORIENTED_EDGE('',*,*,#13193,.F.);
#17290=ORIENTED_EDGE('',*,*,#13350,.T.);
#17291=ORIENTED_EDGE('',*,*,#13351,.T.);
#17292=ORIENTED_EDGE('',*,*,#13280,.T.);
#17293=ORIENTED_EDGE('',*,*,#13297,.F.);
#17294=ORIENTED_EDGE('',*,*,#13299,.F.);
#17295=ORIENTED_EDGE('',*,*,#13301,.F.);
#17296=ORIENTED_EDGE('',*,*,#13303,.F.);
#17297=ORIENTED_EDGE('',*,*,#13305,.F.);
#17298=ORIENTED_EDGE('',*,*,#13307,.T.);
#17299=ORIENTED_EDGE('',*,*,#13309,.T.);
#17300=ORIENTED_EDGE('',*,*,#13339,.T.);
#17301=ORIENTED_EDGE('',*,*,#13225,.F.);
#17302=ORIENTED_EDGE('',*,*,#13228,.T.);
#17303=ORIENTED_EDGE('',*,*,#13213,.F.);
#17304=ORIENTED_EDGE('',*,*,#13341,.T.);
#17305=ORIENTED_EDGE('',*,*,#13274,.T.);
#17306=ORIENTED_EDGE('',*,*,#13028,.T.);
#17307=ORIENTED_EDGE('',*,*,#13022,.T.);
#17308=ORIENTED_EDGE('',*,*,#13254,.F.);
#17309=ORIENTED_EDGE('',*,*,#13265,.F.);
#17310=ORIENTED_EDGE('',*,*,#13421,.F.);
#17311=ORIENTED_EDGE('',*,*,#13422,.F.);
#17312=ORIENTED_EDGE('',*,*,#13237,.F.);
#17313=ORIENTED_EDGE('',*,*,#13248,.F.);
#17314=ORIENTED_EDGE('',*,*,#13423,.F.);
#17315=ORIENTED_EDGE('',*,*,#13424,.F.);
#17316=ORIENTED_EDGE('',*,*,#13232,.F.);
#17317=ORIENTED_EDGE('',*,*,#13425,.F.);
#17318=ORIENTED_EDGE('',*,*,#13323,.F.);
#17319=ORIENTED_EDGE('',*,*,#13426,.T.);
#17320=ORIENTED_EDGE('',*,*,#13359,.F.);
#17321=ORIENTED_EDGE('',*,*,#13336,.F.);
#17322=ORIENTED_EDGE('',*,*,#13326,.F.);
#17323=ORIENTED_EDGE('',*,*,#13233,.T.);
#17324=ORIENTED_EDGE('',*,*,#13229,.F.);
#17325=ORIENTED_EDGE('',*,*,#13425,.T.);
#17326=ORIENTED_EDGE('',*,*,#13231,.F.);
#17327=ORIENTED_EDGE('',*,*,#13235,.T.);
#17328=ORIENTED_EDGE('',*,*,#13245,.F.);
#17329=ORIENTED_EDGE('',*,*,#13424,.T.);
#17330=ORIENTED_EDGE('',*,*,#13427,.T.);
#17331=ORIENTED_EDGE('',*,*,#13251,.F.);
#17332=ORIENTED_EDGE('',*,*,#13262,.F.);
#17333=ORIENTED_EDGE('',*,*,#13422,.T.);
#17334=ORIENTED_EDGE('',*,*,#13428,.T.);
#17335=ORIENTED_EDGE('',*,*,#13268,.F.);
#17336=ORIENTED_EDGE('',*,*,#13421,.T.);
#17337=ORIENTED_EDGE('',*,*,#13264,.T.);
#17338=ORIENTED_EDGE('',*,*,#13267,.F.);
#17339=ORIENTED_EDGE('',*,*,#13269,.F.);
#17340=ORIENTED_EDGE('',*,*,#13428,.F.);
#17341=ORIENTED_EDGE('',*,*,#13423,.T.);
#17342=ORIENTED_EDGE('',*,*,#13247,.T.);
#17343=ORIENTED_EDGE('',*,*,#13250,.F.);
#17344=ORIENTED_EDGE('',*,*,#13252,.F.);
#17345=ORIENTED_EDGE('',*,*,#13427,.F.);
#17346=ORIENTED_EDGE('',*,*,#13320,.F.);
#17347=ORIENTED_EDGE('',*,*,#13329,.T.);
#17348=ORIENTED_EDGE('',*,*,#13362,.F.);
#17349=ORIENTED_EDGE('',*,*,#13429,.F.);
#17350=ORIENTED_EDGE('',*,*,#13322,.F.);
#17351=ORIENTED_EDGE('',*,*,#13429,.T.);
#17352=ORIENTED_EDGE('',*,*,#13361,.F.);
#17353=ORIENTED_EDGE('',*,*,#13426,.F.);
#23550=CONICAL_SURFACE('',#25108,8.75,0.785398163397447);
#23551=CONICAL_SURFACE('',#25115,8.75,0.785398163397447);
#23552=CONICAL_SURFACE('',#25122,10.25,0.785398163397449);
#23553=CONICAL_SURFACE('',#25130,10.25,0.785398163397448);
#23554=CONICAL_SURFACE('',#25168,5.3,0.785398163397446);
#23555=CONICAL_SURFACE('',#25172,5.3,0.785398163397446);
#23556=CONICAL_SURFACE('',#25190,5.3,0.785398163397446);
#23557=CONICAL_SURFACE('',#25206,5.3,0.785398163397446);
#23558=CONICAL_SURFACE('',#25207,5.3,0.785398163397446);
#23559=CONICAL_SURFACE('',#25208,5.3,0.785398163397446);
#23560=CONICAL_SURFACE('',#25209,5.75,0.785398163397446);
#23561=CONICAL_SURFACE('',#25213,5.75,0.785398163397446);
#23562=CONICAL_SURFACE('',#25223,5.75,0.785398163397447);
#23563=CONICAL_SURFACE('',#25224,5.75,0.785398163397447);
#23564=CONICAL_SURFACE('',#25226,1.25,0.785398163397465);
#23565=CONICAL_SURFACE('',#25230,1.25,0.785398163397454);
#23606=ADVANCED_FACE('',(#1747),#23550,.T.);
#23607=ADVANCED_FACE('',(#1748,#586),#711,.F.);
#23608=ADVANCED_FACE('',(#1749),#400,.T.);
#23609=ADVANCED_FACE('',(#1750),#23551,.T.);
#23610=ADVANCED_FACE('',(#1751,#587),#712,.F.);
#23611=ADVANCED_FACE('',(#1752),#401,.T.);
#23612=ADVANCED_FACE('',(#1753),#23552,.F.);
#23613=ADVANCED_FACE('',(#1754),#402,.F.);
#23614=ADVANCED_FACE('',(#1755,#588),#713,.F.);
#23615=ADVANCED_FACE('',(#1756),#23553,.F.);
#23616=ADVANCED_FACE('',(#1757,#589),#714,.T.);
#23617=ADVANCED_FACE('',(#1758),#390,.T.);
#23618=ADVANCED_FACE('',(#1759),#391,.T.);
#23619=ADVANCED_FACE('',(#1760),#715,.T.);
#23620=ADVANCED_FACE('',(#1761,#590,#591,#592,#593,#594,#595),#716,.F.);
#23621=ADVANCED_FACE('',(#1762),#403,.T.);
#23622=ADVANCED_FACE('',(#1763),#717,.T.);
#23623=ADVANCED_FACE('',(#1764),#392,.T.);
#23624=ADVANCED_FACE('',(#1765),#393,.T.);
#23625=ADVANCED_FACE('',(#1766),#718,.T.);
#23626=ADVANCED_FACE('',(#1767),#404,.T.);
#23627=ADVANCED_FACE('',(#1768),#719,.T.);
#23628=ADVANCED_FACE('',(#1769),#23554,.F.);
#23629=ADVANCED_FACE('',(#1770),#405,.F.);
#23630=ADVANCED_FACE('',(#1771),#23555,.F.);
#23631=ADVANCED_FACE('',(#1772),#406,.F.);
#23632=ADVANCED_FACE('',(#1773),#720,.T.);
#23633=ADVANCED_FACE('',(#1774),#407,.F.);
#23634=ADVANCED_FACE('',(#1775),#721,.T.);
#23635=ADVANCED_FACE('',(#1776),#408,.F.);
#23636=ADVANCED_FACE('',(#1777),#722,.T.);
#23637=ADVANCED_FACE('',(#1778),#723,.T.);
#23638=ADVANCED_FACE('',(#1779),#23556,.F.);
#23639=ADVANCED_FACE('',(#1780,#596,#597,#598,#599,#600,#601,#602,#603,
#604),#724,.T.);
#23640=ADVANCED_FACE('',(#1781),#23557,.F.);
#23641=ADVANCED_FACE('',(#1782),#23558,.F.);
#23642=ADVANCED_FACE('',(#1783),#23559,.F.);
#23643=ADVANCED_FACE('',(#1784),#23560,.F.);
#23644=ADVANCED_FACE('',(#1785),#409,.F.);
#23645=ADVANCED_FACE('',(#1786),#23561,.F.);
#23646=ADVANCED_FACE('',(#1787),#410,.F.);
#23647=ADVANCED_FACE('',(#1788),#394,.T.);
#23648=ADVANCED_FACE('',(#1789),#395,.T.);
#23649=ADVANCED_FACE('',(#1790),#725,.T.);
#23650=ADVANCED_FACE('',(#1791),#411,.T.);
#23651=ADVANCED_FACE('',(#1792),#726,.T.);
#23652=ADVANCED_FACE('',(#1793),#396,.T.);
#23653=ADVANCED_FACE('',(#1794),#397,.T.);
#23654=ADVANCED_FACE('',(#1795),#727,.T.);
#23655=ADVANCED_FACE('',(#1796),#412,.T.);
#23656=ADVANCED_FACE('',(#1797),#728,.T.);
#23657=ADVANCED_FACE('',(#1798),#23562,.F.);
#23658=ADVANCED_FACE('',(#1799),#23563,.F.);
#23659=ADVANCED_FACE('',(#1800),#729,.T.);
#23660=ADVANCED_FACE('',(#1801),#23564,.T.);
#23661=ADVANCED_FACE('',(#1802),#730,.T.);
#23662=ADVANCED_FACE('',(#1803),#23565,.T.);
#23663=ADVANCED_FACE('',(#1804),#731,.T.);
#23664=ADVANCED_FACE('',(#1805),#732,.T.);
#23665=ADVANCED_FACE('',(#1806),#192,.T.);
#23666=ADVANCED_FACE('',(#1807),#413,.T.);
#23667=ADVANCED_FACE('',(#1808),#193,.T.);
#23668=ADVANCED_FACE('',(#1809),#194,.T.);
#23669=ADVANCED_FACE('',(#1810),#195,.T.);
#23670=ADVANCED_FACE('',(#1811),#414,.T.);
#23671=ADVANCED_FACE('',(#1812),#415,.T.);
#23672=ADVANCED_FACE('',(#1813),#416,.T.);
#23673=ADVANCED_FACE('',(#1814),#733,.F.);
#23674=ADVANCED_FACE('',(#1815),#417,.F.);
#23675=ADVANCED_FACE('',(#1816),#196,.T.);
#23676=ADVANCED_FACE('',(#1817),#197,.T.);
#23677=ADVANCED_FACE('',(#1818),#198,.T.);
#23678=ADVANCED_FACE('',(#1819),#418,.T.);
#23679=ADVANCED_FACE('',(#1820),#419,.T.);
#23680=ADVANCED_FACE('',(#1821),#420,.T.);
#23681=ADVANCED_FACE('',(#1822),#734,.F.);
#23682=ADVANCED_FACE('',(#1823),#421,.F.);
#23683=ADVANCED_FACE('',(#1824),#199,.T.);
#23684=ADVANCED_FACE('',(#1825),#200,.T.);
#23685=ADVANCED_FACE('',(#1826),#422,.T.);
#23686=ADVANCED_FACE('',(#1827),#201,.T.);
#23687=ADVANCED_FACE('',(#1828),#423,.T.);
#23688=ADVANCED_FACE('',(#1829),#424,.T.);
#23689=ADVANCED_FACE('',(#1830),#202,.T.);
#23690=ADVANCED_FACE('',(#1831),#203,.T.);
#23691=ADVANCED_FACE('',(#1832),#204,.T.);
#23692=ADVANCED_FACE('',(#1833),#425,.T.);
#23693=ADVANCED_FACE('',(#1834),#205,.T.);
#23694=ADVANCED_FACE('',(#1835),#426,.T.);
#23695=ADVANCED_FACE('',(#1836),#735,.F.);
#23696=ADVANCED_FACE('',(#1837),#427,.F.);
#23697=ADVANCED_FACE('',(#1838),#736,.F.);
#23698=ADVANCED_FACE('',(#1839),#428,.F.);
#23699=ADVANCED_FACE('',(#1840),#737,.F.);
#23700=ADVANCED_FACE('',(#1841),#429,.T.);
#23701=ADVANCED_FACE('',(#1842),#430,.T.);
#23702=ADVANCED_FACE('',(#1843),#431,.T.);
#23703=ADVANCED_FACE('',(#1844),#206,.T.);
#23704=ADVANCED_FACE('',(#1845),#432,.T.);
#23705=ADVANCED_FACE('',(#1846),#207,.T.);
#23706=ADVANCED_FACE('',(#1847),#433,.T.);
#23707=ADVANCED_FACE('',(#1848),#208,.T.);
#23708=ADVANCED_FACE('',(#1849),#434,.T.);
#23709=ADVANCED_FACE('',(#1850),#209,.T.);
#23710=ADVANCED_FACE('',(#1851),#435,.T.);
#23711=ADVANCED_FACE('',(#1852),#436,.T.);
#23712=ADVANCED_FACE('',(#1853),#738,.T.);
#23713=ADVANCED_FACE('',(#1854),#437,.T.);
#23714=ADVANCED_FACE('',(#1855),#739,.T.);
#23715=ADVANCED_FACE('',(#1856),#438,.T.);
#23716=ADVANCED_FACE('',(#1857),#439,.T.);
#23717=ADVANCED_FACE('',(#1858),#740,.T.);
#23718=ADVANCED_FACE('',(#1859),#440,.T.);
#23719=ADVANCED_FACE('',(#1860),#741,.T.);
#23720=ADVANCED_FACE('',(#1861),#210,.T.);
#23721=ADVANCED_FACE('',(#1862),#441,.T.);
#23722=ADVANCED_FACE('',(#1863),#211,.T.);
#23723=ADVANCED_FACE('',(#1864),#442,.T.);
#23724=ADVANCED_FACE('',(#1865),#742,.T.);
#23725=ADVANCED_FACE('',(#1866),#443,.T.);
#23726=ADVANCED_FACE('',(#1867),#212,.T.);
#23727=ADVANCED_FACE('',(#1868),#444,.T.);
#23728=ADVANCED_FACE('',(#1869),#213,.T.);
#23729=ADVANCED_FACE('',(#1870),#445,.T.);
#23730=ADVANCED_FACE('',(#1871),#214,.T.);
#23731=ADVANCED_FACE('',(#1872),#446,.T.);
#23732=ADVANCED_FACE('',(#1873),#215,.T.);
#23733=ADVANCED_FACE('',(#1874),#447,.T.);
#23734=ADVANCED_FACE('',(#1875),#216,.T.);
#23735=ADVANCED_FACE('',(#1876),#448,.T.);
#23736=ADVANCED_FACE('',(#1877,#605),#743,.T.);
#23737=ADVANCED_FACE('',(#1878),#449,.T.);
#23738=ADVANCED_FACE('',(#1879),#744,.T.);
#23739=ADVANCED_FACE('',(#1880),#217,.T.);
#23740=ADVANCED_FACE('',(#1881),#218,.T.);
#23741=ADVANCED_FACE('',(#1882),#745,.T.);
#23742=ADVANCED_FACE('',(#1883),#219,.T.);
#23743=ADVANCED_FACE('',(#1884),#220,.T.);
#23744=ADVANCED_FACE('',(#1885),#746,.T.);
#23745=ADVANCED_FACE('',(#1886),#450,.T.);
#23746=ADVANCED_FACE('',(#1887),#221,.T.);
#23747=ADVANCED_FACE('',(#1888),#451,.T.);
#23748=ADVANCED_FACE('',(#1889),#222,.T.);
#23749=ADVANCED_FACE('',(#1890),#452,.F.);
#23750=ADVANCED_FACE('',(#1891),#747,.F.);
#23751=ADVANCED_FACE('',(#1892),#453,.T.);
#23752=ADVANCED_FACE('',(#1893),#223,.T.);
#23753=ADVANCED_FACE('',(#1894),#454,.T.);
#23754=ADVANCED_FACE('',(#1895),#224,.T.);
#23755=ADVANCED_FACE('',(#1896),#455,.T.);
#23756=ADVANCED_FACE('',(#1897),#748,.F.);
#23757=ADVANCED_FACE('',(#1898),#456,.T.);
#23758=ADVANCED_FACE('',(#1899),#749,.F.);
#23759=ADVANCED_FACE('',(#1900),#457,.F.);
#23760=ADVANCED_FACE('',(#1901),#750,.F.);
#23761=ADVANCED_FACE('',(#1902,#606),#751,.T.);
#23762=ADVANCED_FACE('',(#1903),#458,.F.);
#23763=ADVANCED_FACE('',(#1904),#752,.T.);
#23764=ADVANCED_FACE('',(#1905),#459,.F.);
#23765=ADVANCED_FACE('',(#1906),#753,.T.);
#23766=ADVANCED_FACE('',(#1907,#607),#754,.F.);
#23767=ADVANCED_FACE('',(#1908),#460,.F.);
#23768=ADVANCED_FACE('',(#1909,#608),#755,.F.);
#23769=ADVANCED_FACE('',(#1910),#461,.F.);
#23770=ADVANCED_FACE('',(#1911),#462,.F.);
#23771=ADVANCED_FACE('',(#1912,#609,#610),#756,.F.);
#23772=ADVANCED_FACE('',(#1913),#463,.T.);
#23773=ADVANCED_FACE('',(#1914),#464,.T.);
#23774=ADVANCED_FACE('',(#1915),#757,.T.);
#23775=ADVANCED_FACE('',(#1916),#758,.T.);
#23776=ADVANCED_FACE('',(#1917),#759,.F.);
#23777=ADVANCED_FACE('',(#1918),#760,.F.);
#23778=ADVANCED_FACE('',(#1919),#761,.F.);
#23779=ADVANCED_FACE('',(#1920),#762,.F.);
#23780=ADVANCED_FACE('',(#1921),#763,.T.);
#23781=ADVANCED_FACE('',(#1922),#465,.T.);
#24937=CLOSED_SHELL('',(#23606,#23607,#23608,#23609,#23610,#23611,#23612,
#23613,#23614,#23615,#23616,#23617,#23618,#23619,#23620,#23621,#23622,#23623,
#23624,#23625,#23626,#23627,#23628,#23629,#23630,#23631,#23632,#23633,#23634,
#23635,#23636,#23637,#23638,#23639,#23640,#23641,#23642,#23643,#23644,#23645,
#23646,#23647,#23648,#23649,#23650,#23651,#23652,#23653,#23654,#23655,#23656,
#23657,#23658,#23659,#23660,#23661,#23662,#23663,#23664,#23665,#23666,#23667,
#23668,#23669,#23670,#23671,#23672,#23673,#23674,#23675,#23676,#23677,#23678,
#23679,#23680,#23681,#23682,#23683,#23684,#23685,#23686,#23687,#23688,#23689,
#23690,#23691,#23692,#23693,#23694,#23695,#23696,#23697,#23698,#23699,#23700,
#23701,#23702,#23703,#23704,#23705,#23706,#23707,#23708,#23709,#23710,#23711,
#23712,#23713,#23714,#23715,#23716,#23717,#23718,#23719,#23720,#23721,#23722,
#23723,#23724,#23725,#23726,#23727,#23728,#23729,#23730,#23731,#23732,#23733,
#23734,#23735,#23736,#23737,#23738,#23739,#23740,#23741,#23742,#23743,#23744,
#23745,#23746,#23747,#23748,#23749,#23750,#23751,#23752,#23753,#23754,#23755,
#23756,#23757,#23758,#23759,#23760,#23761,#23762,#23763,#23764,#23765,#23766,
#23767,#23768,#23769,#23770,#23771,#23772,#23773,#23774,#23775,#23776,#23777,
#23778,#23779,#23780,#23781));
#25107=AXIS2_PLACEMENT_3D('',#33457,#26935,#26936);
#25108=AXIS2_PLACEMENT_3D('',#33458,#26937,#26938);
#25109=AXIS2_PLACEMENT_3D('',#33460,#26939,#26940);
#25110=AXIS2_PLACEMENT_3D('',#33463,#26942,#26943);
#25111=AXIS2_PLACEMENT_3D('',#33464,#26944,#26945);
#25112=AXIS2_PLACEMENT_3D('',#33466,#26946,#26947);
#25113=AXIS2_PLACEMENT_3D('',#33467,#26948,#26949);
#25114=AXIS2_PLACEMENT_3D('',#33470,#26951,#26952);
#25115=AXIS2_PLACEMENT_3D('',#33471,#26953,#26954);
#25116=AXIS2_PLACEMENT_3D('',#33473,#26955,#26956);
#25117=AXIS2_PLACEMENT_3D('',#33476,#26958,#26959);
#25118=AXIS2_PLACEMENT_3D('',#33477,#26960,#26961);
#25119=AXIS2_PLACEMENT_3D('',#33479,#26962,#26963);
#25120=AXIS2_PLACEMENT_3D('',#33480,#26964,#26965);
#25121=AXIS2_PLACEMENT_3D('',#33483,#26967,#26968);
#25122=AXIS2_PLACEMENT_3D('',#33484,#26969,#26970);
#25123=AXIS2_PLACEMENT_3D('',#33486,#26971,#26972);
#25124=AXIS2_PLACEMENT_3D('',#33490,#26974,#26975);
#25125=AXIS2_PLACEMENT_3D('',#33491,#26976,#26977);
#25126=AXIS2_PLACEMENT_3D('',#33492,#26978,#26979);
#25127=AXIS2_PLACEMENT_3D('',#33495,#26981,#26982);
#25128=AXIS2_PLACEMENT_3D('',#33496,#26983,#26984);
#25129=AXIS2_PLACEMENT_3D('',#33498,#26985,#26986);
#25130=AXIS2_PLACEMENT_3D('',#33499,#26987,#26988);
#25131=AXIS2_PLACEMENT_3D('',#33501,#26989,#26990);
#25132=AXIS2_PLACEMENT_3D('',#33503,#26992,#26993);
#25133=AXIS2_PLACEMENT_3D('',#33508,#26995,#26996);
#25134=AXIS2_PLACEMENT_3D('',#33511,#26998,#26999);
#25135=AXIS2_PLACEMENT_3D('',#33694,#27002,#27003);
#25136=AXIS2_PLACEMENT_3D('',#33700,#27007,#27008);
#25137=AXIS2_PLACEMENT_3D('',#33705,#27010,#27011);
#25138=AXIS2_PLACEMENT_3D('',#33709,#27013,#27014);
#25139=AXIS2_PLACEMENT_3D('',#33713,#27016,#27017);
#25140=AXIS2_PLACEMENT_3D('',#33717,#27019,#27020);
#25141=AXIS2_PLACEMENT_3D('',#33720,#27022,#27023);
#25142=AXIS2_PLACEMENT_3D('',#33722,#27024,#27025);
#25143=AXIS2_PLACEMENT_3D('',#33730,#27029,#27030);
#25144=AXIS2_PLACEMENT_3D('',#33738,#27034,#27035);
#25145=AXIS2_PLACEMENT_3D('',#33740,#27036,#27037);
#25146=AXIS2_PLACEMENT_3D('',#33744,#27039,#27040);
#25147=AXIS2_PLACEMENT_3D('',#33748,#27042,#27043);
#25148=AXIS2_PLACEMENT_3D('',#33752,#27045,#27046);
#25149=AXIS2_PLACEMENT_3D('',#33754,#27047,#27048);
#25150=AXIS2_PLACEMENT_3D('',#33766,#27054,#27055);
#25151=AXIS2_PLACEMENT_3D('',#33770,#27057,#27058);
#25152=AXIS2_PLACEMENT_3D('',#33774,#27060,#27061);
#25153=AXIS2_PLACEMENT_3D('',#33776,#27062,#27063);
#25154=AXIS2_PLACEMENT_3D('',#33780,#27065,#27066);
#25155=AXIS2_PLACEMENT_3D('',#33782,#27067,#27068);
#25156=AXIS2_PLACEMENT_3D('',#33784,#27069,#27070);
#25157=AXIS2_PLACEMENT_3D('',#33786,#27071,#27072);
#25158=AXIS2_PLACEMENT_3D('',#33787,#27073,#27074);
#25159=AXIS2_PLACEMENT_3D('',#33790,#27075,#27076);
#25160=AXIS2_PLACEMENT_3D('',#33794,#27078,#27079);
#25161=AXIS2_PLACEMENT_3D('',#33796,#27080,#27081);
#25162=AXIS2_PLACEMENT_3D('',#33799,#27083,#27084);
#25163=AXIS2_PLACEMENT_3D('',#33800,#27085,#27086);
#25164=AXIS2_PLACEMENT_3D('',#33866,#27088,#27089);
#25165=AXIS2_PLACEMENT_3D('',#33991,#27093,#27094);
#25166=AXIS2_PLACEMENT_3D('',#33995,#27097,#27098);
#25167=AXIS2_PLACEMENT_3D('',#34012,#27100,#27101);
#25168=AXIS2_PLACEMENT_3D('',#34016,#27104,#27105);
#25169=AXIS2_PLACEMENT_3D('',#34019,#27107,#27108);
#25170=AXIS2_PLACEMENT_3D('',#34020,#27109,#27110);
#25171=AXIS2_PLACEMENT_3D('',#34022,#27111,#27112);
#25172=AXIS2_PLACEMENT_3D('',#34024,#27114,#27115);
#25173=AXIS2_PLACEMENT_3D('',#34027,#27117,#27118);
#25174=AXIS2_PLACEMENT_3D('',#34028,#27119,#27120);
#25175=AXIS2_PLACEMENT_3D('',#34030,#27121,#27122);
#25176=AXIS2_PLACEMENT_3D('',#34032,#27124,#27125);
#25177=AXIS2_PLACEMENT_3D('',#34051,#27128,#27129);
#25178=AXIS2_PLACEMENT_3D('',#34053,#27130,#27131);
#25179=AXIS2_PLACEMENT_3D('',#34057,#27133,#27134);
#25180=AXIS2_PLACEMENT_3D('',#34067,#27135,#27136);
#25181=AXIS2_PLACEMENT_3D('',#34079,#27138,#27139);
#25182=AXIS2_PLACEMENT_3D('',#34080,#27140,#27141);
#25183=AXIS2_PLACEMENT_3D('',#34099,#27144,#27145);
#25184=AXIS2_PLACEMENT_3D('',#34101,#27146,#27147);
#25185=AXIS2_PLACEMENT_3D('',#34104,#27149,#27150);
#25186=AXIS2_PLACEMENT_3D('',#34115,#27151,#27152);
#25187=AXIS2_PLACEMENT_3D('',#34127,#27154,#27155);
#25188=AXIS2_PLACEMENT_3D('',#34128,#27156,#27157);
#25189=AXIS2_PLACEMENT_3D('',#34144,#27159,#27160);
#25190=AXIS2_PLACEMENT_3D('',#34160,#27162,#27163);
#25191=AXIS2_PLACEMENT_3D('',#34162,#27164,#27165);
#25192=AXIS2_PLACEMENT_3D('',#34164,#27167,#27168);
#25193=AXIS2_PLACEMENT_3D('',#34167,#27169,#27170);
#25194=AXIS2_PLACEMENT_3D('',#34171,#27172,#27173);
#25195=AXIS2_PLACEMENT_3D('',#34175,#27175,#27176);
#25196=AXIS2_PLACEMENT_3D('',#34179,#27178,#27179);
#25197=AXIS2_PLACEMENT_3D('',#34182,#27181,#27182);
#25198=AXIS2_PLACEMENT_3D('',#34184,#27183,#27184);
#25199=AXIS2_PLACEMENT_3D('',#34186,#27185,#27186);
#25200=AXIS2_PLACEMENT_3D('',#34191,#27188,#27189);
#25201=AXIS2_PLACEMENT_3D('',#34194,#27191,#27192);
#25202=AXIS2_PLACEMENT_3D('',#34196,#27193,#27194);
#25203=AXIS2_PLACEMENT_3D('',#34198,#27195,#27196);
#25204=AXIS2_PLACEMENT_3D('',#34200,#27197,#27198);
#25205=AXIS2_PLACEMENT_3D('',#34202,#27199,#27200);
#25206=AXIS2_PLACEMENT_3D('',#34203,#27201,#27202);
#25207=AXIS2_PLACEMENT_3D('',#34205,#27204,#27205);
#25208=AXIS2_PLACEMENT_3D('',#34207,#27207,#27208);
#25209=AXIS2_PLACEMENT_3D('',#34209,#27210,#27211);
#25210=AXIS2_PLACEMENT_3D('',#34212,#27213,#27214);
#25211=AXIS2_PLACEMENT_3D('',#34213,#27215,#27216);
#25212=AXIS2_PLACEMENT_3D('',#34215,#27217,#27218);
#25213=AXIS2_PLACEMENT_3D('',#34217,#27220,#27221);
#25214=AXIS2_PLACEMENT_3D('',#34220,#27223,#27224);
#25215=AXIS2_PLACEMENT_3D('',#34221,#27225,#27226);
#25216=AXIS2_PLACEMENT_3D('',#34223,#27227,#27228);
#25217=AXIS2_PLACEMENT_3D('',#34404,#27231,#27232);
#25218=AXIS2_PLACEMENT_3D('',#34410,#27236,#27237);
#25219=AXIS2_PLACEMENT_3D('',#34475,#27239,#27240);
#25220=AXIS2_PLACEMENT_3D('',#34595,#27244,#27245);
#25221=AXIS2_PLACEMENT_3D('',#34599,#27248,#27249);
#25222=AXIS2_PLACEMENT_3D('',#34616,#27251,#27252);
#25223=AXIS2_PLACEMENT_3D('',#34620,#27255,#27256);
#25224=AXIS2_PLACEMENT_3D('',#34622,#27258,#27259);
#25225=AXIS2_PLACEMENT_3D('',#34624,#27261,#27262);
#25226=AXIS2_PLACEMENT_3D('',#34633,#27267,#27268);
#25227=AXIS2_PLACEMENT_3D('',#34636,#27270,#27271);
#25228=AXIS2_PLACEMENT_3D('',#34637,#27272,#27273);
#25229=AXIS2_PLACEMENT_3D('',#34638,#27274,#27275);
#25230=AXIS2_PLACEMENT_3D('',#34642,#27278,#27279);
#25231=AXIS2_PLACEMENT_3D('',#34646,#27281,#27282);
#25232=AXIS2_PLACEMENT_3D('',#34647,#27283,#27284);
#25233=AXIS2_PLACEMENT_3D('',#34648,#27285,#27286);
#25234=AXIS2_PLACEMENT_3D('',#34654,#27290,#27291);
#25235=AXIS2_PLACEMENT_3D('',#34656,#27293,#27294);
#25236=AXIS2_PLACEMENT_3D('',#34672,#27295,#27296);
#25237=AXIS2_PLACEMENT_3D('',#34686,#27297,#27298);
#25238=AXIS2_PLACEMENT_3D('',#34687,#27299,#27300);
#25239=AXIS2_PLACEMENT_3D('',#34691,#27302,#27303);
#25240=AXIS2_PLACEMENT_3D('',#34693,#27305,#27306);
#25241=AXIS2_PLACEMENT_3D('',#34710,#27307,#27308);
#25242=AXIS2_PLACEMENT_3D('',#34725,#27309,#27310);
#25243=AXIS2_PLACEMENT_3D('',#34741,#27311,#27312);
#25244=AXIS2_PLACEMENT_3D('',#34742,#27313,#27314);
#25245=AXIS2_PLACEMENT_3D('',#34744,#27315,#27316);
#25246=AXIS2_PLACEMENT_3D('',#34746,#27317,#27318);
#25247=AXIS2_PLACEMENT_3D('',#34747,#27319,#27320);
#25248=AXIS2_PLACEMENT_3D('',#34748,#27321,#27322);
#25249=AXIS2_PLACEMENT_3D('',#34750,#27324,#27325);
#25250=AXIS2_PLACEMENT_3D('',#34752,#27327,#27328);
#25251=AXIS2_PLACEMENT_3D('',#34756,#27330,#27331);
#25252=AXIS2_PLACEMENT_3D('',#34758,#27333,#27334);
#25253=AXIS2_PLACEMENT_3D('',#34762,#27337,#27338);
#25254=AXIS2_PLACEMENT_3D('',#34765,#27340,#27341);
#25255=AXIS2_PLACEMENT_3D('',#34766,#27342,#27343);
#25256=AXIS2_PLACEMENT_3D('',#34783,#27344,#27345);
#25257=AXIS2_PLACEMENT_3D('',#34798,#27346,#27347);
#25258=AXIS2_PLACEMENT_3D('',#34814,#27348,#27349);
#25259=AXIS2_PLACEMENT_3D('',#34815,#27350,#27351);
#25260=AXIS2_PLACEMENT_3D('',#34817,#27352,#27353);
#25261=AXIS2_PLACEMENT_3D('',#34819,#27354,#27355);
#25262=AXIS2_PLACEMENT_3D('',#34820,#27356,#27357);
#25263=AXIS2_PLACEMENT_3D('',#34821,#27358,#27359);
#25264=AXIS2_PLACEMENT_3D('',#34823,#27361,#27362);
#25265=AXIS2_PLACEMENT_3D('',#34825,#27364,#27365);
#25266=AXIS2_PLACEMENT_3D('',#34829,#27367,#27368);
#25267=AXIS2_PLACEMENT_3D('',#34831,#27370,#27371);
#25268=AXIS2_PLACEMENT_3D('',#34835,#27374,#27375);
#25269=AXIS2_PLACEMENT_3D('',#34838,#27377,#27378);
#25270=AXIS2_PLACEMENT_3D('',#34839,#27379,#27380);
#25271=AXIS2_PLACEMENT_3D('',#34868,#27381,#27382);
#25272=AXIS2_PLACEMENT_3D('',#34870,#27383,#27384);
#25273=AXIS2_PLACEMENT_3D('',#34885,#27385,#27386);
#25274=AXIS2_PLACEMENT_3D('',#34887,#27387,#27388);
#25275=AXIS2_PLACEMENT_3D('',#34889,#27390,#27391);
#25276=AXIS2_PLACEMENT_3D('',#34906,#27392,#27393);
#25277=AXIS2_PLACEMENT_3D('',#34921,#27394,#27395);
#25278=AXIS2_PLACEMENT_3D('',#34925,#27397,#27398);
#25279=AXIS2_PLACEMENT_3D('',#34927,#27400,#27401);
#25280=AXIS2_PLACEMENT_3D('',#34931,#27403,#27404);
#25281=AXIS2_PLACEMENT_3D('',#34946,#27405,#27406);
#25282=AXIS2_PLACEMENT_3D('',#34962,#27407,#27408);
#25283=AXIS2_PLACEMENT_3D('',#34963,#27409,#27410);
#25284=AXIS2_PLACEMENT_3D('',#34979,#27411,#27412);
#25285=AXIS2_PLACEMENT_3D('',#34980,#27413,#27414);
#25286=AXIS2_PLACEMENT_3D('',#34982,#27415,#27416);
#25287=AXIS2_PLACEMENT_3D('',#34983,#27417,#27418);
#25288=AXIS2_PLACEMENT_3D('',#34984,#27419,#27420);
#25289=AXIS2_PLACEMENT_3D('',#34986,#27421,#27422);
#25290=AXIS2_PLACEMENT_3D('',#34988,#27424,#27425);
#25291=AXIS2_PLACEMENT_3D('',#34990,#27426,#27427);
#25292=AXIS2_PLACEMENT_3D('',#34991,#27428,#27429);
#25293=AXIS2_PLACEMENT_3D('',#34992,#27430,#27431);
#25294=AXIS2_PLACEMENT_3D('',#34994,#27433,#27434);
#25295=AXIS2_PLACEMENT_3D('',#34998,#27437,#27438);
#25296=AXIS2_PLACEMENT_3D('',#35001,#27440,#27441);
#25297=AXIS2_PLACEMENT_3D('',#35002,#27442,#27443);
#25298=AXIS2_PLACEMENT_3D('',#35006,#27446,#27447);
#25299=AXIS2_PLACEMENT_3D('',#35009,#27449,#27450);
#25300=AXIS2_PLACEMENT_3D('',#35010,#27451,#27452);
#25301=AXIS2_PLACEMENT_3D('',#35014,#27455,#27456);
#25302=AXIS2_PLACEMENT_3D('',#35017,#27458,#27459);
#25303=AXIS2_PLACEMENT_3D('',#35018,#27460,#27461);
#25304=AXIS2_PLACEMENT_3D('',#35021,#27463,#27464);
#25305=AXIS2_PLACEMENT_3D('',#35022,#27465,#27466);
#25306=AXIS2_PLACEMENT_3D('',#35024,#27467,#27468);
#25307=AXIS2_PLACEMENT_3D('',#35027,#27470,#27471);
#25308=AXIS2_PLACEMENT_3D('',#35028,#27472,#27473);
#25309=AXIS2_PLACEMENT_3D('',#35030,#27474,#27475);
#25310=AXIS2_PLACEMENT_3D('',#35031,#27476,#27477);
#25311=AXIS2_PLACEMENT_3D('',#35032,#27478,#27479);
#25312=AXIS2_PLACEMENT_3D('',#35034,#27480,#27481);
#25313=AXIS2_PLACEMENT_3D('',#35036,#27483,#27484);
#25314=AXIS2_PLACEMENT_3D('',#35038,#27485,#27486);
#25315=AXIS2_PLACEMENT_3D('',#35039,#27487,#27488);
#25316=AXIS2_PLACEMENT_3D('',#35040,#27489,#27490);
#25317=AXIS2_PLACEMENT_3D('',#35042,#27491,#27492);
#25318=AXIS2_PLACEMENT_3D('',#35044,#27494,#27495);
#25319=AXIS2_PLACEMENT_3D('',#35046,#27496,#27497);
#25320=AXIS2_PLACEMENT_3D('',#35047,#27498,#27499);
#25321=AXIS2_PLACEMENT_3D('',#35048,#27500,#27501);
#25322=AXIS2_PLACEMENT_3D('',#35050,#27503,#27504);
#25323=AXIS2_PLACEMENT_3D('',#35052,#27505,#27506);
#25324=AXIS2_PLACEMENT_3D('',#35053,#27507,#27508);
#25325=AXIS2_PLACEMENT_3D('',#35054,#27509,#27510);
#25326=AXIS2_PLACEMENT_3D('',#35056,#27512,#27513);
#25327=AXIS2_PLACEMENT_3D('',#35060,#27515,#27516);
#25328=AXIS2_PLACEMENT_3D('',#35062,#27518,#27519);
#25329=AXIS2_PLACEMENT_3D('',#35066,#27522,#27523);
#25330=AXIS2_PLACEMENT_3D('',#35069,#27525,#27526);
#25331=AXIS2_PLACEMENT_3D('',#35070,#27527,#27528);
#25332=AXIS2_PLACEMENT_3D('',#35074,#27531,#27532);
#25333=AXIS2_PLACEMENT_3D('',#35077,#27534,#27535);
#25334=AXIS2_PLACEMENT_3D('',#35078,#27536,#27537);
#25335=AXIS2_PLACEMENT_3D('',#35080,#27539,#27540);
#25336=AXIS2_PLACEMENT_3D('',#35082,#27542,#27543);
#25337=AXIS2_PLACEMENT_3D('',#35084,#27545,#27546);
#25338=AXIS2_PLACEMENT_3D('',#35086,#27548,#27549);
#25339=AXIS2_PLACEMENT_3D('',#35088,#27550,#27551);
#25340=AXIS2_PLACEMENT_3D('',#35103,#27552,#27553);
#25341=AXIS2_PLACEMENT_3D('',#35120,#27555,#27556);
#25342=AXIS2_PLACEMENT_3D('',#35121,#27557,#27558);
#25343=AXIS2_PLACEMENT_3D('',#35122,#27559,#27560);
#25344=AXIS2_PLACEMENT_3D('',#35124,#27561,#27562);
#25345=AXIS2_PLACEMENT_3D('',#35126,#27564,#27565);
#25346=AXIS2_PLACEMENT_3D('',#35130,#27568,#27569);
#25347=AXIS2_PLACEMENT_3D('',#35131,#27570,#27571);
#25348=AXIS2_PLACEMENT_3D('',#35132,#27572,#27573);
#25349=AXIS2_PLACEMENT_3D('',#35133,#27574,#27575);
#25350=AXIS2_PLACEMENT_3D('',#35134,#27576,#27577);
#25351=AXIS2_PLACEMENT_3D('',#35135,#27578,#27579);
#25352=AXIS2_PLACEMENT_3D('',#35136,#27580,#27581);
#25353=AXIS2_PLACEMENT_3D('',#35137,#27582,#27583);
#25354=AXIS2_PLACEMENT_3D('',#35138,#27584,#27585);
#25355=AXIS2_PLACEMENT_3D('',#35139,#27586,#27587);
#25356=AXIS2_PLACEMENT_3D('',#35140,#27588,#27589);
#25357=AXIS2_PLACEMENT_3D('',#35141,#27590,#27591);
#25358=AXIS2_PLACEMENT_3D('',#35142,#27592,#27593);
#25359=AXIS2_PLACEMENT_3D('',#35143,#27594,#27595);
#25360=AXIS2_PLACEMENT_3D('',#35145,#27596,#27597);
#25361=AXIS2_PLACEMENT_3D('',#35147,#27599,#27600);
#25362=AXIS2_PLACEMENT_3D('',#35149,#27601,#27602);
#25363=AXIS2_PLACEMENT_3D('',#35150,#27603,#27604);
#25364=AXIS2_PLACEMENT_3D('',#35151,#27605,#27606);
#25365=AXIS2_PLACEMENT_3D('',#35153,#27608,#27609);
#25366=AXIS2_PLACEMENT_3D('',#35155,#27610,#27611);
#25367=AXIS2_PLACEMENT_3D('',#35157,#27612,#27613);
#25368=AXIS2_PLACEMENT_3D('',#35158,#27614,#27615);
#25369=AXIS2_PLACEMENT_3D('',#35159,#27616,#27617);
#25370=AXIS2_PLACEMENT_3D('',#35160,#27618,#27619);
#25371=AXIS2_PLACEMENT_3D('',#35175,#27620,#27621);
#25372=AXIS2_PLACEMENT_3D('',#35191,#27623,#27624);
#25373=AXIS2_PLACEMENT_3D('',#35193,#27625,#27626);
#25374=AXIS2_PLACEMENT_3D('',#35194,#27627,#27628);
#25375=AXIS2_PLACEMENT_3D('',#35196,#27630,#27631);
#25376=AXIS2_PLACEMENT_3D('',#35198,#27633,#27634);
#25377=AXIS2_PLACEMENT_3D('',#35199,#27635,#27636);
#25378=AXIS2_PLACEMENT_3D('',#35200,#27637,#27638);
#25379=AXIS2_PLACEMENT_3D('',#35201,#27639,#27640);
#25380=AXIS2_PLACEMENT_3D('',#35202,#27641,#27642);
#25381=AXIS2_PLACEMENT_3D('',#35203,#27643,#27644);
#25382=AXIS2_PLACEMENT_3D('',#35204,#27645,#27646);
#25383=AXIS2_PLACEMENT_3D('',#35205,#27647,#27648);
#25384=AXIS2_PLACEMENT_3D('',#35206,#27649,#27650);
#25385=AXIS2_PLACEMENT_3D('',#35208,#27651,#27652);
#25386=AXIS2_PLACEMENT_3D('',#35211,#27654,#27655);
#25387=AXIS2_PLACEMENT_3D('',#35212,#27656,#27657);
#25388=AXIS2_PLACEMENT_3D('',#35214,#27658,#27659);
#25389=AXIS2_PLACEMENT_3D('',#35215,#27660,#27661);
#25390=AXIS2_PLACEMENT_3D('',#35216,#27662,#27663);
#25391=AXIS2_PLACEMENT_3D('',#35218,#27664,#27665);
#25392=AXIS2_PLACEMENT_3D('',#35220,#27667,#27668);
#25393=AXIS2_PLACEMENT_3D('',#35221,#27669,#27670);
#25394=AXIS2_PLACEMENT_3D('',#35222,#27671,#27672);
#25395=AXIS2_PLACEMENT_3D('',#35226,#27674,#27675);
#25396=AXIS2_PLACEMENT_3D('',#35228,#27677,#27678);
#25397=AXIS2_PLACEMENT_3D('',#35232,#27681,#27682);
#25398=AXIS2_PLACEMENT_3D('',#35234,#27683,#27684);
#25399=AXIS2_PLACEMENT_3D('',#35237,#27686,#27687);
#25400=AXIS2_PLACEMENT_3D('',#35238,#27688,#27689);
#25401=AXIS2_PLACEMENT_3D('',#35240,#27690,#27691);
#25402=AXIS2_PLACEMENT_3D('',#35241,#27692,#27693);
#25403=AXIS2_PLACEMENT_3D('',#35242,#27694,#27695);
#25404=AXIS2_PLACEMENT_3D('',#35244,#27696,#27697);
#25405=AXIS2_PLACEMENT_3D('',#35246,#27699,#27700);
#25406=AXIS2_PLACEMENT_3D('',#35247,#27701,#27702);
#25407=AXIS2_PLACEMENT_3D('',#35248,#27703,#27704);
#25408=AXIS2_PLACEMENT_3D('',#35252,#27706,#27707);
#25409=AXIS2_PLACEMENT_3D('',#35254,#27709,#27710);
#25410=AXIS2_PLACEMENT_3D('',#35258,#27713,#27714);
#25411=AXIS2_PLACEMENT_3D('',#35261,#27716,#27717);
#25412=AXIS2_PLACEMENT_3D('',#35262,#27718,#27719);
#25413=AXIS2_PLACEMENT_3D('',#35264,#27721,#27722);
#25414=AXIS2_PLACEMENT_3D('',#35267,#27724,#27725);
#25415=AXIS2_PLACEMENT_3D('',#35268,#27726,#27727);
#25416=AXIS2_PLACEMENT_3D('',#35270,#27729,#27730);
#25417=AXIS2_PLACEMENT_3D('',#35271,#27731,#27732);
#25418=AXIS2_PLACEMENT_3D('',#35274,#27734,#27735);
#25419=AXIS2_PLACEMENT_3D('',#35275,#27736,#27737);
#25420=AXIS2_PLACEMENT_3D('',#35276,#27738,#27739);
#25421=AXIS2_PLACEMENT_3D('',#35279,#27741,#27742);
#25422=AXIS2_PLACEMENT_3D('',#35280,#27743,#27744);
#25423=AXIS2_PLACEMENT_3D('',#35281,#27745,#27746);
#25424=AXIS2_PLACEMENT_3D('',#35283,#27747,#27748);
#25425=AXIS2_PLACEMENT_3D('',#35285,#27749,#27750);
#25426=AXIS2_PLACEMENT_3D('',#35286,#27751,#27752);
#25427=AXIS2_PLACEMENT_3D('',#35289,#27754,#27755);
#25428=AXIS2_PLACEMENT_3D('',#35290,#27756,#27757);
#25429=AXIS2_PLACEMENT_3D('',#35292,#27758,#27759);
#25430=AXIS2_PLACEMENT_3D('',#35293,#27760,#27761);
#25431=AXIS2_PLACEMENT_3D('',#35295,#27763,#27764);
#25432=AXIS2_PLACEMENT_3D('',#35297,#27766,#27767);
#25433=AXIS2_PLACEMENT_3D('',#35298,#27768,#27769);
#25434=AXIS2_PLACEMENT_3D('',#35300,#27770,#27771);
#25435=AXIS2_PLACEMENT_3D('',#35302,#27773,#27774);
#25436=AXIS2_PLACEMENT_3D('',#35304,#27775,#27776);
#25437=AXIS2_PLACEMENT_3D('',#35306,#27778,#27779);
#25438=AXIS2_PLACEMENT_3D('',#35308,#27781,#27782);
#25439=AXIS2_PLACEMENT_3D('',#35310,#27784,#27785);
#25440=AXIS2_PLACEMENT_3D('',#35312,#27787,#27788);
#25441=AXIS2_PLACEMENT_3D('',#35314,#27790,#27791);
#25442=AXIS2_PLACEMENT_3D('',#35315,#27792,#27793);
#25443=AXIS2_PLACEMENT_3D('',#35316,#27794,#27795);
#25444=AXIS2_PLACEMENT_3D('',#35318,#27797,#27798);
#26935=DIRECTION('axis',(0.,0.,1.));
#26936=DIRECTION('refdir',(1.,0.,0.));
#26937=DIRECTION('center_axis',(0.,1.,0.));
#26938=DIRECTION('ref_axis',(1.,0.,0.));
#26939=DIRECTION('center_axis',(0.,1.,0.));
#26940=DIRECTION('ref_axis',(1.,0.,0.));
#26941=DIRECTION('',(-0.707106781186547,0.707106781186549,-8.65956056235492E-17));
#26942=DIRECTION('center_axis',(0.,-1.,0.));
#26943=DIRECTION('ref_axis',(1.,0.,0.));
#26944=DIRECTION('center_axis',(0.,1.,0.));
#26945=DIRECTION('ref_axis',(1.,0.,0.));
#26946=DIRECTION('center_axis',(0.,-1.,0.));
#26947=DIRECTION('ref_axis',(1.,0.,0.));
#26948=DIRECTION('center_axis',(0.,-1.,0.));
#26949=DIRECTION('ref_axis',(1.,0.,0.));
#26950=DIRECTION('',(0.,1.,0.));
#26951=DIRECTION('center_axis',(0.,1.,0.));
#26952=DIRECTION('ref_axis',(1.,0.,0.));
#26953=DIRECTION('center_axis',(0.,1.,0.));
#26954=DIRECTION('ref_axis',(1.,0.,0.));
#26955=DIRECTION('center_axis',(0.,1.,0.));
#26956=DIRECTION('ref_axis',(1.,0.,0.));
#26957=DIRECTION('',(-0.707106781186547,0.707106781186549,-8.65956056235492E-17));
#26958=DIRECTION('center_axis',(0.,-1.,0.));
#26959=DIRECTION('ref_axis',(1.,0.,0.));
#26960=DIRECTION('center_axis',(0.,1.,0.));
#26961=DIRECTION('ref_axis',(1.,0.,0.));
#26962=DIRECTION('center_axis',(0.,-1.,0.));
#26963=DIRECTION('ref_axis',(1.,0.,0.));
#26964=DIRECTION('center_axis',(0.,-1.,0.));
#26965=DIRECTION('ref_axis',(1.,0.,0.));
#26966=DIRECTION('',(0.,1.,0.));
#26967=DIRECTION('center_axis',(0.,1.,0.));
#26968=DIRECTION('ref_axis',(1.,0.,0.));
#26969=DIRECTION('center_axis',(0.,-1.,0.));
#26970=DIRECTION('ref_axis',(0.,0.,-1.));
#26971=DIRECTION('center_axis',(0.,-1.,0.));
#26972=DIRECTION('ref_axis',(0.,0.,-1.));
#26973=DIRECTION('',(8.65956056235494E-17,0.707106781186547,-0.707106781186548));
#26974=DIRECTION('center_axis',(0.,1.,0.));
#26975=DIRECTION('ref_axis',(0.,0.,-1.));
#26976=DIRECTION('center_axis',(0.,1.,0.));
#26977=DIRECTION('ref_axis',(0.,0.,-1.));
#26978=DIRECTION('center_axis',(0.,1.,0.));
#26979=DIRECTION('ref_axis',(0.,0.,1.));
#26980=DIRECTION('',(0.,1.,0.));
#26981=DIRECTION('center_axis',(0.,-1.,0.));
#26982=DIRECTION('ref_axis',(0.,0.,1.));
#26983=DIRECTION('center_axis',(0.,1.,0.));
#26984=DIRECTION('ref_axis',(0.,0.,1.));
#26985=DIRECTION('center_axis',(0.,1.,0.));
#26986=DIRECTION('ref_axis',(1.,0.,0.));
#26987=DIRECTION('center_axis',(0.,1.,0.));
#26988=DIRECTION('ref_axis',(0.,0.,1.));
#26989=DIRECTION('center_axis',(0.,1.,0.));
#26990=DIRECTION('ref_axis',(0.,0.,1.));
#26991=DIRECTION('',(8.65956056235493E-17,-0.707106781186548,0.707106781186548));
#26992=DIRECTION('center_axis',(0.,1.,0.));
#26993=DIRECTION('ref_axis',(1.,0.,0.));
#26994=DIRECTION('',(0.,0.,-1.));
#26995=DIRECTION('center_axis',(0.,-1.,0.));
#26996=DIRECTION('ref_axis',(-6.12323399573676E-17,0.,1.));
#26997=DIRECTION('',(0.,0.,1.));
#26998=DIRECTION('center_axis',(0.,-1.,0.));
#26999=DIRECTION('ref_axis',(8.54643792476272E-17,0.,-1.));
#27000=DIRECTION('',(-0.707106781186549,0.,0.707106781186546));
#27001=DIRECTION('',(0.707106781186551,0.,-0.707106781186544));
#27002=DIRECTION('center_axis',(-0.707106781186547,0.,-0.707106781186548));
#27003=DIRECTION('ref_axis',(-0.707106781186548,0.,0.707106781186547));
#27004=DIRECTION('',(-0.707106781186548,0.,0.707106781186547));
#27005=DIRECTION('',(0.,-1.,0.));
#27006=DIRECTION('',(0.,1.,0.));
#27007=DIRECTION('center_axis',(0.,1.,0.));
#27008=DIRECTION('ref_axis',(1.,0.,0.));
#27009=DIRECTION('',(1.,0.,0.));
#27010=DIRECTION('center_axis',(0.,1.,0.));
#27011=DIRECTION('ref_axis',(-0.707106781186547,0.,0.707106781186547));
#27012=DIRECTION('',(0.,0.,1.));
#27013=DIRECTION('center_axis',(0.,1.,0.));
#27014=DIRECTION('ref_axis',(-0.707106781186547,0.,-0.707106781186547));
#27015=DIRECTION('',(-1.,0.,0.));
#27016=DIRECTION('center_axis',(0.,1.,0.));
#27017=DIRECTION('ref_axis',(0.707106781186548,0.,-0.707106781186547));
#27018=DIRECTION('',(0.,0.,-1.));
#27019=DIRECTION('center_axis',(0.,1.,0.));
#27020=DIRECTION('ref_axis',(0.707106781186547,0.,0.707106781186548));
#27021=DIRECTION('',(1.,0.,0.));
#27022=DIRECTION('center_axis',(0.,1.,0.));
#27023=DIRECTION('ref_axis',(6.12323399573677E-17,0.,1.));
#27024=DIRECTION('center_axis',(0.,-1.,0.));
#27025=DIRECTION('ref_axis',(1.,0.,0.));
#27026=DIRECTION('',(-1.,0.,0.));
#27027=DIRECTION('',(-0.707106781186549,0.,-0.707106781186546));
#27028=DIRECTION('',(5.04646829375071E-17,0.,-1.));
#27029=DIRECTION('center_axis',(0.,1.,0.));
#27030=DIRECTION('ref_axis',(0.38268343236509,0.,-0.923879532511287));
#27031=DIRECTION('',(-0.707106781186548,0.,0.707106781186548));
#27032=DIRECTION('',(-0.707106781186548,0.,-0.707106781186548));
#27033=DIRECTION('',(0.707106781186548,0.,-0.707106781186548));
#27034=DIRECTION('center_axis',(0.,1.,0.));
#27035=DIRECTION('ref_axis',(0.892598706858255,0.,-0.450852025075824));
#27036=DIRECTION('center_axis',(0.,1.,0.));
#27037=DIRECTION('ref_axis',(-0.117423234417673,0.,-0.99308196238724));
#27038=DIRECTION('',(0.,0.,1.));
#27039=DIRECTION('center_axis',(0.,-1.,0.));
#27040=DIRECTION('ref_axis',(0.707106781186547,0.,-0.707106781186548));
#27041=DIRECTION('',(1.,0.,0.));
#27042=DIRECTION('center_axis',(0.,-1.,0.));
#27043=DIRECTION('ref_axis',(-0.707106781186548,0.,-0.707106781186548));
#27044=DIRECTION('',(0.,0.,-1.));
#27045=DIRECTION('center_axis',(0.,1.,0.));
#27046=DIRECTION('ref_axis',(0.12088535091488,0.,-0.992666475677599));
#27047=DIRECTION('center_axis',(0.,1.,0.));
#27048=DIRECTION('ref_axis',(-0.899687500253878,0.,-0.436534536877586));
#27049=DIRECTION('',(0.707106781186548,0.,0.707106781186547));
#27050=DIRECTION('',(8.91235409254052E-15,0.,1.));
#27051=DIRECTION('',(-0.707106781186548,0.,0.707106781186547));
#27052=DIRECTION('',(-1.,0.,-8.91235409254068E-15));
#27053=DIRECTION('',(-0.707106781186548,0.,-0.707106781186548));
#27054=DIRECTION('center_axis',(0.,1.,0.));
#27055=DIRECTION('ref_axis',(-0.367874908669274,0.,-0.929875288182008));
#27056=DIRECTION('',(-5.04646829375071E-17,0.,1.));
#27057=DIRECTION('center_axis',(0.,-1.,0.));
#27058=DIRECTION('ref_axis',(0.707106781186548,0.,0.707106781186547));
#27059=DIRECTION('',(0.,0.,1.));
#27060=DIRECTION('center_axis',(0.,1.,0.));
#27061=DIRECTION('ref_axis',(-0.117423234417673,0.,0.99308196238724));
#27062=DIRECTION('center_axis',(0.,1.,0.));
#27063=DIRECTION('ref_axis',(0.868290222566564,0.,0.496056538506759));
#27064=DIRECTION('',(-1.,0.,0.));
#27065=DIRECTION('center_axis',(0.,-1.,0.));
#27066=DIRECTION('ref_axis',(0.811029676142761,0.,0.585005012299696));
#27067=DIRECTION('center_axis',(0.,1.,0.));
#27068=DIRECTION('ref_axis',(0.,0.,1.));
#27069=DIRECTION('center_axis',(0.,1.,0.));
#27070=DIRECTION('ref_axis',(0.,0.,1.));
#27071=DIRECTION('center_axis',(0.,-1.,0.));
#27072=DIRECTION('ref_axis',(-0.811029676142761,0.,0.585005012299696));
#27073=DIRECTION('center_axis',(0.,1.,0.));
#27074=DIRECTION('ref_axis',(0.,0.,1.));
#27075=DIRECTION('center_axis',(0.,-1.,0.));
#27076=DIRECTION('ref_axis',(-0.707106781186547,0.,0.707106781186548));
#27077=DIRECTION('',(-1.,0.,0.));
#27078=DIRECTION('center_axis',(0.,1.,0.));
#27079=DIRECTION('ref_axis',(-0.868290222566564,0.,0.496056538506759));
#27080=DIRECTION('center_axis',(0.,1.,0.));
#27081=DIRECTION('ref_axis',(0.117423234417673,0.,0.99308196238724));
#27082=DIRECTION('',(0.,0.,-1.));
#27083=DIRECTION('center_axis',(0.,-1.,0.));
#27084=DIRECTION('ref_axis',(1.,0.,0.));
#27085=DIRECTION('center_axis',(1.,0.,0.));
#27086=DIRECTION('ref_axis',(0.,-0.707106781186547,-0.707106781186548));
#27087=DIRECTION('',(1.,0.,0.));
#27088=DIRECTION('center_axis',(0.,0.,-1.));
#27089=DIRECTION('ref_axis',(1.,0.,0.));
#27090=DIRECTION('',(-1.,0.,0.));
#27091=DIRECTION('',(0.,1.,0.));
#27092=DIRECTION('',(0.707106781186548,0.,0.707106781186547));
#27093=DIRECTION('center_axis',(0.707106781186553,0.,-0.707106781186542));
#27094=DIRECTION('ref_axis',(-0.707106781186542,0.,-0.707106781186553));
#27095=DIRECTION('',(-0.707106781186542,0.,-0.707106781186553));
#27096=DIRECTION('',(0.,-1.,0.));
#27097=DIRECTION('center_axis',(-5.04646829375071E-17,0.,1.));
#27098=DIRECTION('ref_axis',(0.707106781186548,-0.707106781186548,0.));
#27099=DIRECTION('',(-5.04646829375071E-17,0.,1.));
#27100=DIRECTION('center_axis',(1.,0.,5.04646829375071E-17));
#27101=DIRECTION('ref_axis',(-5.04646829375071E-17,0.,1.));
#27102=DIRECTION('',(5.04646829375071E-17,0.,-1.));
#27103=DIRECTION('',(0.,1.,0.));
#27104=DIRECTION('center_axis',(0.,-1.,0.));
#27105=DIRECTION('ref_axis',(1.,0.,0.));
#27106=DIRECTION('',(0.707106781186546,0.707106781186549,8.65956056235491E-17));
#27107=DIRECTION('center_axis',(0.,1.,0.));
#27108=DIRECTION('ref_axis',(1.,0.,0.));
#27109=DIRECTION('center_axis',(0.,-1.,0.));
#27110=DIRECTION('ref_axis',(1.,0.,0.));
#27111=DIRECTION('center_axis',(0.,-1.,0.));
#27112=DIRECTION('ref_axis',(1.,0.,0.));
#27113=DIRECTION('',(0.,-1.,0.));
#27114=DIRECTION('center_axis',(0.,-1.,0.));
#27115=DIRECTION('ref_axis',(1.,0.,0.));
#27116=DIRECTION('',(0.707106781186546,0.707106781186549,8.65956056235491E-17));
#27117=DIRECTION('center_axis',(0.,1.,0.));
#27118=DIRECTION('ref_axis',(1.,0.,0.));
#27119=DIRECTION('center_axis',(0.,-1.,0.));
#27120=DIRECTION('ref_axis',(1.,0.,0.));
#27121=DIRECTION('center_axis',(0.,-1.,0.));
#27122=DIRECTION('ref_axis',(1.,0.,0.));
#27123=DIRECTION('',(0.,-1.,0.));
#27124=DIRECTION('center_axis',(-0.15189042169011,0.,0.988397339028592));
#27125=DIRECTION('ref_axis',(0.988397339028592,0.,0.15189042169011));
#27126=DIRECTION('',(0.,-1.,0.));
#27127=DIRECTION('',(0.,1.,0.));
#27128=DIRECTION('center_axis',(0.,-1.,0.));
#27129=DIRECTION('ref_axis',(1.,0.,0.));
#27130=DIRECTION('center_axis',(0.,-1.,0.));
#27131=DIRECTION('ref_axis',(1.,0.,0.));
#27132=DIRECTION('',(0.,-1.,0.));
#27133=DIRECTION('center_axis',(0.,-1.,0.));
#27134=DIRECTION('ref_axis',(1.,0.,0.));
#27135=DIRECTION('center_axis',(0.,1.,0.));
#27136=DIRECTION('ref_axis',(0.811029676142761,0.,0.585005012299696));
#27137=DIRECTION('',(0.,1.,0.));
#27138=DIRECTION('center_axis',(0.,-1.,0.));
#27139=DIRECTION('ref_axis',(1.,0.,0.));
#27140=DIRECTION('center_axis',(0.15189042169011,0.,0.988397339028592));
#27141=DIRECTION('ref_axis',(0.988397339028592,0.,-0.15189042169011));
#27142=DIRECTION('',(0.,1.,0.));
#27143=DIRECTION('',(0.,-1.,0.));
#27144=DIRECTION('center_axis',(0.,-1.,0.));
#27145=DIRECTION('ref_axis',(1.,0.,0.));
#27146=DIRECTION('center_axis',(0.,-1.,0.));
#27147=DIRECTION('ref_axis',(1.,0.,0.));
#27148=DIRECTION('',(0.,-1.,0.));
#27149=DIRECTION('center_axis',(0.,1.,0.));
#27150=DIRECTION('ref_axis',(-0.811029676142761,0.,0.585005012299696));
#27151=DIRECTION('center_axis',(0.,-1.,0.));
#27152=DIRECTION('ref_axis',(1.,0.,0.));
#27153=DIRECTION('',(0.,-1.,0.));
#27154=DIRECTION('center_axis',(0.,1.,0.));
#27155=DIRECTION('ref_axis',(-0.811029676142761,0.,0.585005012299696));
#27156=DIRECTION('center_axis',(-0.889975696162041,0.,-0.456007960720962));
#27157=DIRECTION('ref_axis',(-0.456007960720962,0.,0.889975696162041));
#27158=DIRECTION('',(0.,1.,0.));
#27159=DIRECTION('center_axis',(0.889975696162041,0.,-0.456007960720962));
#27160=DIRECTION('ref_axis',(-0.456007960720962,0.,-0.889975696162041));
#27161=DIRECTION('',(0.,-1.,0.));
#27162=DIRECTION('center_axis',(0.,1.,0.));
#27163=DIRECTION('ref_axis',(1.,0.,0.));
#27164=DIRECTION('center_axis',(0.,1.,0.));
#27165=DIRECTION('ref_axis',(1.,0.,0.));
#27166=DIRECTION('',(0.707106781186546,-0.707106781186549,-8.65956056235491E-17));
#27167=DIRECTION('center_axis',(0.,1.,0.));
#27168=DIRECTION('ref_axis',(1.,0.,0.));
#27169=DIRECTION('center_axis',(0.,-1.,0.));
#27170=DIRECTION('ref_axis',(0.707106781186548,0.,-0.707106781186547));
#27171=DIRECTION('',(1.,0.,0.));
#27172=DIRECTION('center_axis',(0.,-1.,0.));
#27173=DIRECTION('ref_axis',(-0.707106781186547,0.,-0.707106781186547));
#27174=DIRECTION('',(0.,0.,-1.));
#27175=DIRECTION('center_axis',(0.,-1.,0.));
#27176=DIRECTION('ref_axis',(-0.707106781186547,0.,0.707106781186547));
#27177=DIRECTION('',(-1.,0.,0.));
#27178=DIRECTION('center_axis',(0.,-1.,0.));
#27179=DIRECTION('ref_axis',(0.707106781186547,0.,0.707106781186548));
#27180=DIRECTION('',(0.,0.,1.));
#27181=DIRECTION('center_axis',(0.,1.,0.));
#27182=DIRECTION('ref_axis',(1.,0.,0.));
#27183=DIRECTION('center_axis',(0.,1.,0.));
#27184=DIRECTION('ref_axis',(1.,0.,0.));
#27185=DIRECTION('center_axis',(0.,1.,0.));
#27186=DIRECTION('ref_axis',(1.,0.,0.));
#27187=DIRECTION('',(0.,0.,-1.));
#27188=DIRECTION('center_axis',(0.,1.,0.));
#27189=DIRECTION('ref_axis',(-6.12323399573676E-17,0.,1.));
#27190=DIRECTION('',(0.,0.,1.));
#27191=DIRECTION('center_axis',(0.,1.,0.));
#27192=DIRECTION('ref_axis',(6.12323399573676E-17,0.,-1.));
#27193=DIRECTION('center_axis',(0.,-1.,0.));
#27194=DIRECTION('ref_axis',(1.,0.,0.));
#27195=DIRECTION('center_axis',(0.,-1.,0.));
#27196=DIRECTION('ref_axis',(1.,0.,0.));
#27197=DIRECTION('center_axis',(0.,1.,0.));
#27198=DIRECTION('ref_axis',(1.,0.,0.));
#27199=DIRECTION('center_axis',(0.,1.,0.));
#27200=DIRECTION('ref_axis',(1.,0.,0.));
#27201=DIRECTION('center_axis',(0.,1.,0.));
#27202=DIRECTION('ref_axis',(1.,0.,0.));
#27203=DIRECTION('',(0.707106781186546,-0.707106781186549,-8.65956056235491E-17));
#27204=DIRECTION('center_axis',(0.,1.,0.));
#27205=DIRECTION('ref_axis',(1.,0.,0.));
#27206=DIRECTION('',(0.707106781186546,-0.707106781186549,-8.65956056235491E-17));
#27207=DIRECTION('center_axis',(0.,1.,0.));
#27208=DIRECTION('ref_axis',(1.,0.,0.));
#27209=DIRECTION('',(0.707106781186546,-0.707106781186549,-8.65956056235491E-17));
#27210=DIRECTION('center_axis',(0.,1.,0.));
#27211=DIRECTION('ref_axis',(1.,0.,0.));
#27212=DIRECTION('',(0.707106781186546,-0.707106781186549,-8.65956056235491E-17));
#27213=DIRECTION('center_axis',(0.,-1.,0.));
#27214=DIRECTION('ref_axis',(1.,0.,0.));
#27215=DIRECTION('center_axis',(0.,1.,0.));
#27216=DIRECTION('ref_axis',(1.,0.,0.));
#27217=DIRECTION('center_axis',(0.,1.,0.));
#27218=DIRECTION('ref_axis',(1.,0.,0.));
#27219=DIRECTION('',(0.,1.,0.));
#27220=DIRECTION('center_axis',(0.,1.,0.));
#27221=DIRECTION('ref_axis',(1.,0.,0.));
#27222=DIRECTION('',(0.707106781186546,-0.707106781186549,-8.65956056235491E-17));
#27223=DIRECTION('center_axis',(0.,-1.,0.));
#27224=DIRECTION('ref_axis',(1.,0.,0.));
#27225=DIRECTION('center_axis',(0.,1.,0.));
#27226=DIRECTION('ref_axis',(1.,0.,0.));
#27227=DIRECTION('center_axis',(0.,1.,0.));
#27228=DIRECTION('ref_axis',(1.,0.,0.));
#27229=DIRECTION('',(0.,1.,0.));
#27230=DIRECTION('',(-1.25607396694705E-14,2.74766180269668E-15,-1.));
#27231=DIRECTION('center_axis',(-1.,0.,0.));
#27232=DIRECTION('ref_axis',(0.,0.,1.));
#27233=DIRECTION('',(0.,0.,1.));
#27234=DIRECTION('',(0.,-1.,0.));
#27235=DIRECTION('',(0.,1.,0.));
#27236=DIRECTION('center_axis',(0.707106781186548,0.,-0.707106781186547));
#27237=DIRECTION('ref_axis',(-0.5,-0.707106781186548,-0.5));
#27238=DIRECTION('',(0.707106781186548,0.,-0.707106781186547));
#27239=DIRECTION('center_axis',(-0.707106781186547,0.,-0.707106781186548));
#27240=DIRECTION('ref_axis',(0.707106781186548,0.,-0.707106781186547));
#27241=DIRECTION('',(-0.707106781186548,0.,0.707106781186547));
#27242=DIRECTION('',(0.,1.,0.));
#27243=DIRECTION('',(1.,0.,-1.25607396694702E-14));
#27244=DIRECTION('center_axis',(0.,0.,-1.));
#27245=DIRECTION('ref_axis',(-1.,0.,0.));
#27246=DIRECTION('',(-1.,0.,0.));
#27247=DIRECTION('',(0.,-1.,0.));
#27248=DIRECTION('center_axis',(0.707106781186548,0.,0.707106781186548));
#27249=DIRECTION('ref_axis',(0.5,-0.707106781186548,-0.5));
#27250=DIRECTION('',(0.707106781186548,0.,0.707106781186548));
#27251=DIRECTION('center_axis',(0.707106781186548,0.,-0.707106781186548));
#27252=DIRECTION('ref_axis',(0.707106781186548,0.,0.707106781186548));
#27253=DIRECTION('',(-0.707106781186548,0.,-0.707106781186548));
#27254=DIRECTION('',(0.,1.,0.));
#27255=DIRECTION('center_axis',(0.,-1.,0.));
#27256=DIRECTION('ref_axis',(1.,0.,0.));
#27257=DIRECTION('',(0.707106781186546,0.707106781186549,8.65956056235492E-17));
#27258=DIRECTION('center_axis',(0.,-1.,0.));
#27259=DIRECTION('ref_axis',(1.,0.,0.));
#27260=DIRECTION('',(0.707106781186546,0.707106781186549,8.65956056235492E-17));
#27261=DIRECTION('center_axis',(0.,0.,-1.));
#27262=DIRECTION('ref_axis',(-1.,0.,0.));
#27263=DIRECTION('',(-1.,0.,0.));
#27264=DIRECTION('',(0.,-1.,0.));
#27265=DIRECTION('',(-1.,0.,0.));
#27266=DIRECTION('',(0.,1.,0.));
#27267=DIRECTION('center_axis',(-0.707106781186548,0.,0.707106781186548));
#27268=DIRECTION('ref_axis',(-0.5,-0.707106781186546,-0.500000000000002));
#27269=DIRECTION('',(-0.499999999999991,-0.707106781186561,0.499999999999991));
#27270=DIRECTION('center_axis',(0.707106781186548,0.,-0.707106781186548));
#27271=DIRECTION('ref_axis',(-0.5,-0.707106781186546,-0.500000000000002));
#27272=DIRECTION('center_axis',(-0.707106781186548,0.,0.707106781186548));
#27273=DIRECTION('ref_axis',(-0.500000000000001,-0.707106781186546,-0.500000000000001));
#27274=DIRECTION('center_axis',(0.5,-0.707106781186547,-0.5));
#27275=DIRECTION('ref_axis',(-0.707106781186548,0.,-0.707106781186548));
#27276=DIRECTION('',(-0.5,-0.707106781186548,0.5));
#27277=DIRECTION('',(0.707106781186548,0.,0.707106781186548));
#27278=DIRECTION('center_axis',(-0.707106781186548,0.,0.707106781186548));
#27279=DIRECTION('ref_axis',(0.499999999999999,-0.707106781186548,0.499999999999999));
#27280=DIRECTION('',(0.,-3.92523114670944E-16,1.));
#27281=DIRECTION('center_axis',(0.707106781186548,0.,-0.707106781186548));
#27282=DIRECTION('ref_axis',(0.5,-0.707106781186548,0.5));
#27283=DIRECTION('center_axis',(-0.707106781186548,0.,0.707106781186548));
#27284=DIRECTION('ref_axis',(0.5,-0.707106781186548,0.5));
#27285=DIRECTION('center_axis',(1.,0.,0.));
#27286=DIRECTION('ref_axis',(0.,0.,-1.));
#27287=DIRECTION('',(0.,0.,-1.));
#27288=DIRECTION('',(0.,-1.,0.));
#27289=DIRECTION('',(0.,1.,0.));
#27290=DIRECTION('center_axis',(0.707106781186548,0.,-0.707106781186548));
#27291=DIRECTION('ref_axis',(0.707106781186548,0.,0.707106781186548));
#27292=DIRECTION('',(-0.707106781186548,0.,-0.707106781186548));
#27293=DIRECTION('center_axis',(0.,1.,0.));
#27294=DIRECTION('ref_axis',(0.,0.,1.));
#27295=DIRECTION('center_axis',(0.,1.,0.));
#27296=DIRECTION('ref_axis',(6.12323399573677E-17,0.,1.));
#27297=DIRECTION('center_axis',(0.,-1.,0.));
#27298=DIRECTION('ref_axis',(6.12323399573677E-17,0.,1.));
#27299=DIRECTION('center_axis',(0.,-1.,0.));
#27300=DIRECTION('ref_axis',(1.,0.,0.));
#27301=DIRECTION('',(0.,1.,0.));
#27302=DIRECTION('center_axis',(0.,-1.,0.));
#27303=DIRECTION('ref_axis',(6.12323399573677E-17,0.,1.));
#27304=DIRECTION('',(0.,-1.,0.));
#27305=DIRECTION('center_axis',(0.,-1.,0.));
#27306=DIRECTION('ref_axis',(0.136763231432696,0.,0.990603764644617));
#27307=DIRECTION('center_axis',(0.,-1.,0.));
#27308=DIRECTION('ref_axis',(0.117423234417673,0.,0.99308196238724));
#27309=DIRECTION('center_axis',(0.,-1.,0.));
#27310=DIRECTION('ref_axis',(0.,0.,-1.));
#27311=DIRECTION('center_axis',(0.,-1.,0.));
#27312=DIRECTION('ref_axis',(-0.868290222566564,0.,0.496056538506759));
#27313=DIRECTION('center_axis',(0.,1.,0.));
#27314=DIRECTION('ref_axis',(0.,0.,1.));
#27315=DIRECTION('center_axis',(-1.48029736616687E-15,0.,1.));
#27316=DIRECTION('ref_axis',(0.,-1.,0.));
#27317=DIRECTION('center_axis',(0.,1.,0.));
#27318=DIRECTION('ref_axis',(-0.707106781186547,0.,0.707106781186548));
#27319=DIRECTION('center_axis',(-1.,0.,0.));
#27320=DIRECTION('ref_axis',(0.,0.,-1.));
#27321=DIRECTION('center_axis',(1.,0.,0.));
#27322=DIRECTION('ref_axis',(0.,-0.707106781186549,-0.707106781186546));
#27323=DIRECTION('',(1.,0.,0.));
#27324=DIRECTION('center_axis',(0.,0.,1.));
#27325=DIRECTION('ref_axis',(0.707106781186548,-0.707106781186547,0.));
#27326=DIRECTION('',(0.,0.,1.));
#27327=DIRECTION('center_axis',(0.,-1.,0.));
#27328=DIRECTION('ref_axis',(1.,0.,0.));
#27329=DIRECTION('',(0.,-1.,0.));
#27330=DIRECTION('center_axis',(0.,1.,0.));
#27331=DIRECTION('ref_axis',(1.,0.,0.));
#27332=DIRECTION('',(0.,-1.,0.));
#27333=DIRECTION('center_axis',(0.,0.,1.));
#27334=DIRECTION('ref_axis',(1.,0.,0.));
#27335=DIRECTION('',(0.,1.,0.));
#27336=DIRECTION('',(1.,0.,0.));
#27337=DIRECTION('center_axis',(0.,1.,0.));
#27338=DIRECTION('ref_axis',(-1.,0.,-1.00929365875014E-16));
#27339=DIRECTION('',(0.,1.,0.));
#27340=DIRECTION('center_axis',(0.,1.,0.));
#27341=DIRECTION('ref_axis',(-1.,0.,-1.00929365875014E-16));
#27342=DIRECTION('center_axis',(0.,-1.,0.));
#27343=DIRECTION('ref_axis',(0.,0.,-1.));
#27344=DIRECTION('center_axis',(0.,-1.,0.));
#27345=DIRECTION('ref_axis',(0.868290222566564,0.,0.496056538506759));
#27346=DIRECTION('center_axis',(0.,-1.,0.));
#27347=DIRECTION('ref_axis',(-0.136763231432696,0.,0.990603764644617));
#27348=DIRECTION('center_axis',(0.,-1.,0.));
#27349=DIRECTION('ref_axis',(-0.117423234417673,0.,0.99308196238724));
#27350=DIRECTION('center_axis',(0.,1.,0.));
#27351=DIRECTION('ref_axis',(0.,0.,1.));
#27352=DIRECTION('center_axis',(1.,0.,2.96059473233376E-15));
#27353=DIRECTION('ref_axis',(0.,-1.,0.));
#27354=DIRECTION('center_axis',(0.,1.,0.));
#27355=DIRECTION('ref_axis',(0.707106781186548,0.,0.707106781186547));
#27356=DIRECTION('center_axis',(0.,0.,1.));
#27357=DIRECTION('ref_axis',(-1.,0.,0.));
#27358=DIRECTION('center_axis',(0.,0.,-1.));
#27359=DIRECTION('ref_axis',(-0.707106781186548,-0.707106781186547,0.));
#27360=DIRECTION('',(0.,0.,-1.));
#27361=DIRECTION('center_axis',(1.,0.,0.));
#27362=DIRECTION('ref_axis',(0.,-0.707106781186549,-0.707106781186546));
#27363=DIRECTION('',(1.,0.,0.));
#27364=DIRECTION('center_axis',(0.,-1.,0.));
#27365=DIRECTION('ref_axis',(1.,0.,0.));
#27366=DIRECTION('',(0.,-1.,0.));
#27367=DIRECTION('center_axis',(0.,1.,0.));
#27368=DIRECTION('ref_axis',(1.,0.,0.));
#27369=DIRECTION('',(0.,-1.,0.));
#27370=DIRECTION('center_axis',(1.,0.,0.));
#27371=DIRECTION('ref_axis',(0.,0.,-1.));
#27372=DIRECTION('',(0.,1.,0.));
#27373=DIRECTION('',(0.,0.,-1.));
#27374=DIRECTION('center_axis',(0.,1.,0.));
#27375=DIRECTION('ref_axis',(2.01858731750029E-16,0.,1.));
#27376=DIRECTION('',(0.,1.,0.));
#27377=DIRECTION('center_axis',(0.,1.,0.));
#27378=DIRECTION('ref_axis',(2.01858731750029E-16,0.,1.));
#27379=DIRECTION('center_axis',(0.,-1.,0.));
#27380=DIRECTION('ref_axis',(1.22464679914735E-16,0.,1.));
#27381=DIRECTION('center_axis',(0.,-1.,0.));
#27382=DIRECTION('ref_axis',(0.,0.,-1.));
#27383=DIRECTION('center_axis',(0.,-1.,0.));
#27384=DIRECTION('ref_axis',(0.38268343236509,0.,-0.923879532511287));
#27385=DIRECTION('center_axis',(0.,-1.,0.));
#27386=DIRECTION('ref_axis',(1.,0.,0.));
#27387=DIRECTION('center_axis',(0.,1.,0.));
#27388=DIRECTION('ref_axis',(1.,0.,0.));
#27389=DIRECTION('',(0.,-1.,0.));
#27390=DIRECTION('center_axis',(0.,-1.,0.));
#27391=DIRECTION('ref_axis',(0.,0.,-1.));
#27392=DIRECTION('center_axis',(0.,-1.,0.));
#27393=DIRECTION('ref_axis',(0.12088535091488,0.,-0.992666475677599));
#27394=DIRECTION('center_axis',(0.,-1.,0.));
#27395=DIRECTION('ref_axis',(1.,0.,0.));
#27396=DIRECTION('',(0.,-1.,0.));
#27397=DIRECTION('center_axis',(0.,1.,0.));
#27398=DIRECTION('ref_axis',(1.,0.,0.));
#27399=DIRECTION('',(0.,-1.,0.));
#27400=DIRECTION('center_axis',(0.,0.,-1.));
#27401=DIRECTION('ref_axis',(-0.707106781186548,-0.707106781186547,0.));
#27402=DIRECTION('',(0.,0.,-1.));
#27403=DIRECTION('center_axis',(0.,0.,1.));
#27404=DIRECTION('ref_axis',(-1.,0.,0.));
#27405=DIRECTION('center_axis',(0.,-1.,0.));
#27406=DIRECTION('ref_axis',(0.,0.,-1.));
#27407=DIRECTION('center_axis',(0.,-1.,0.));
#27408=DIRECTION('ref_axis',(-0.117423234417673,0.,-0.99308196238724));
#27409=DIRECTION('center_axis',(0.,-1.,0.));
#27410=DIRECTION('ref_axis',(0.,0.,-1.));
#27411=DIRECTION('center_axis',(0.,-1.,0.));
#27412=DIRECTION('ref_axis',(0.892598706858255,0.,-0.450852025075824));
#27413=DIRECTION('center_axis',(0.,1.,0.));
#27414=DIRECTION('ref_axis',(0.,0.,1.));
#27415=DIRECTION('center_axis',(1.,0.,-2.96059473233378E-15));
#27416=DIRECTION('ref_axis',(2.96059473233378E-15,0.,1.));
#27417=DIRECTION('center_axis',(0.,1.,0.));
#27418=DIRECTION('ref_axis',(0.707106781186547,0.,-0.707106781186548));
#27419=DIRECTION('center_axis',(-1.,0.,0.));
#27420=DIRECTION('ref_axis',(0.,-0.707106781186547,0.707106781186548));
#27421=DIRECTION('center_axis',(1.,0.,-2.96059473233374E-15));
#27422=DIRECTION('ref_axis',(2.96059473233374E-15,0.,1.));
#27423=DIRECTION('',(-1.,0.,0.));
#27424=DIRECTION('center_axis',(0.,1.,0.));
#27425=DIRECTION('ref_axis',(0.,0.,1.));
#27426=DIRECTION('center_axis',(0.,0.,-1.));
#27427=DIRECTION('ref_axis',(1.,0.,0.));
#27428=DIRECTION('center_axis',(0.,1.,0.));
#27429=DIRECTION('ref_axis',(-0.707106781186547,0.,-0.707106781186547));
#27430=DIRECTION('center_axis',(0.,0.,1.));
#27431=DIRECTION('ref_axis',(0.707106781186548,-0.707106781186547,0.));
#27432=DIRECTION('',(0.,0.,1.));
#27433=DIRECTION('center_axis',(-1.,0.,0.));
#27434=DIRECTION('ref_axis',(0.,0.,1.));
#27435=DIRECTION('',(0.,1.,0.));
#27436=DIRECTION('',(0.,0.,1.));
#27437=DIRECTION('center_axis',(0.,1.,0.));
#27438=DIRECTION('ref_axis',(2.01858731750029E-16,0.,-1.));
#27439=DIRECTION('',(0.,1.,0.));
#27440=DIRECTION('center_axis',(0.,1.,0.));
#27441=DIRECTION('ref_axis',(2.01858731750029E-16,0.,-1.));
#27442=DIRECTION('center_axis',(0.,0.,-1.));
#27443=DIRECTION('ref_axis',(-1.,0.,0.));
#27444=DIRECTION('',(0.,1.,0.));
#27445=DIRECTION('',(-1.,0.,0.));
#27446=DIRECTION('center_axis',(0.,1.,0.));
#27447=DIRECTION('ref_axis',(1.,0.,8.07434927000114E-16));
#27448=DIRECTION('',(0.,1.,0.));
#27449=DIRECTION('center_axis',(0.,1.,0.));
#27450=DIRECTION('ref_axis',(1.,0.,8.07434927000114E-16));
#27451=DIRECTION('center_axis',(1.,0.,0.));
#27452=DIRECTION('ref_axis',(0.,0.,-1.));
#27453=DIRECTION('',(0.,1.,0.));
#27454=DIRECTION('',(0.,0.,-1.));
#27455=DIRECTION('center_axis',(0.,-1.,0.));
#27456=DIRECTION('ref_axis',(1.,0.,0.));
#27457=DIRECTION('',(0.,-1.,0.));
#27458=DIRECTION('center_axis',(0.,1.,0.));
#27459=DIRECTION('ref_axis',(1.,0.,0.));
#27460=DIRECTION('center_axis',(0.,-1.,0.));
#27461=DIRECTION('ref_axis',(1.,0.,0.));
#27462=DIRECTION('',(0.,1.,0.));
#27463=DIRECTION('center_axis',(0.,1.,0.));
#27464=DIRECTION('ref_axis',(1.,0.,0.));
#27465=DIRECTION('center_axis',(0.,0.,-1.));
#27466=DIRECTION('ref_axis',(-0.707106781186548,-0.707106781186547,0.));
#27467=DIRECTION('center_axis',(-1.48029736616687E-15,0.,-1.));
#27468=DIRECTION('ref_axis',(0.,-1.,0.));
#27469=DIRECTION('',(0.,0.,-1.));
#27470=DIRECTION('center_axis',(0.,0.,1.));
#27471=DIRECTION('ref_axis',(-1.,0.,0.));
#27472=DIRECTION('center_axis',(0.,1.,0.));
#27473=DIRECTION('ref_axis',(0.,0.,1.));
#27474=DIRECTION('center_axis',(-1.,0.,0.));
#27475=DIRECTION('ref_axis',(0.,0.,-1.));
#27476=DIRECTION('center_axis',(0.,-1.,0.));
#27477=DIRECTION('ref_axis',(-0.707106781186548,0.,-0.707106781186548));
#27478=DIRECTION('center_axis',(1.,0.,0.));
#27479=DIRECTION('ref_axis',(0.,-0.707106781186547,-0.707106781186548));
#27480=DIRECTION('center_axis',(-1.,0.,0.));
#27481=DIRECTION('ref_axis',(0.,0.,-1.));
#27482=DIRECTION('',(1.,0.,0.));
#27483=DIRECTION('center_axis',(0.,1.,0.));
#27484=DIRECTION('ref_axis',(0.,0.,1.));
#27485=DIRECTION('center_axis',(0.,0.,-1.));
#27486=DIRECTION('ref_axis',(1.,0.,0.));
#27487=DIRECTION('center_axis',(0.,-1.,0.));
#27488=DIRECTION('ref_axis',(0.707106781186548,0.,-0.707106781186547));
#27489=DIRECTION('center_axis',(0.,0.,1.));
#27490=DIRECTION('ref_axis',(0.707106781186548,-0.707106781186547,0.));
#27491=DIRECTION('center_axis',(0.,0.,-1.));
#27492=DIRECTION('ref_axis',(1.,0.,0.));
#27493=DIRECTION('',(0.,0.,1.));
#27494=DIRECTION('center_axis',(0.,1.,0.));
#27495=DIRECTION('ref_axis',(0.,0.,1.));
#27496=DIRECTION('center_axis',(1.,0.,-5.92118946466749E-15));
#27497=DIRECTION('ref_axis',(5.92118946466749E-15,0.,1.));
#27498=DIRECTION('center_axis',(0.,-1.,0.));
#27499=DIRECTION('ref_axis',(0.707106781186547,0.,0.707106781186548));
#27500=DIRECTION('center_axis',(-1.,0.,0.));
#27501=DIRECTION('ref_axis',(0.,-0.707106781186547,0.707106781186548));
#27502=DIRECTION('',(-1.,0.,0.));
#27503=DIRECTION('center_axis',(0.,1.,0.));
#27504=DIRECTION('ref_axis',(0.,0.,1.));
#27505=DIRECTION('center_axis',(-1.,0.,0.));
#27506=DIRECTION('ref_axis',(0.,-1.,0.));
#27507=DIRECTION('center_axis',(0.,-1.,0.));
#27508=DIRECTION('ref_axis',(-0.707106781186548,0.,0.707106781186548));
#27509=DIRECTION('center_axis',(-1.,0.,0.));
#27510=DIRECTION('ref_axis',(0.,-0.707106781186547,0.707106781186548));
#27511=DIRECTION('',(-1.,0.,0.));
#27512=DIRECTION('center_axis',(0.,1.,0.));
#27513=DIRECTION('ref_axis',(1.,0.,0.));
#27514=DIRECTION('',(0.,1.,0.));
#27515=DIRECTION('center_axis',(0.,1.,0.));
#27516=DIRECTION('ref_axis',(0.707106781186548,0.,-0.707106781186547));
#27517=DIRECTION('',(0.,1.,0.));
#27518=DIRECTION('center_axis',(0.,0.,-1.));
#27519=DIRECTION('ref_axis',(-1.,0.,0.));
#27520=DIRECTION('',(0.,1.,0.));
#27521=DIRECTION('',(-1.,0.,0.));
#27522=DIRECTION('center_axis',(0.,1.,0.));
#27523=DIRECTION('ref_axis',(-3.1720657846433E-16,0.,-1.));
#27524=DIRECTION('',(0.,1.,0.));
#27525=DIRECTION('center_axis',(0.,1.,0.));
#27526=DIRECTION('ref_axis',(-0.707106781186548,0.,-0.707106781186548));
#27527=DIRECTION('center_axis',(-1.,0.,0.));
#27528=DIRECTION('ref_axis',(0.,0.,1.));
#27529=DIRECTION('',(0.,1.,0.));
#27530=DIRECTION('',(0.,0.,1.));
#27531=DIRECTION('center_axis',(0.,1.,0.));
#27532=DIRECTION('ref_axis',(-1.,0.,3.96508223080413E-16));
#27533=DIRECTION('',(0.,1.,0.));
#27534=DIRECTION('center_axis',(0.,1.,0.));
#27535=DIRECTION('ref_axis',(-0.707106781186548,0.,0.707106781186548));
#27536=DIRECTION('center_axis',(-0.707106781186548,0.,0.707106781186548));
#27537=DIRECTION('ref_axis',(0.5,-0.707106781186548,0.5));
#27538=DIRECTION('',(-0.707106781186548,0.,0.707106781186548));
#27539=DIRECTION('center_axis',(0.707106781186548,0.,0.707106781186548));
#27540=DIRECTION('ref_axis',(-0.707106781186548,0.,0.707106781186548));
#27541=DIRECTION('',(0.707106781186548,0.,-0.707106781186548));
#27542=DIRECTION('center_axis',(0.707106781186548,0.,-0.707106781186548));
#27543=DIRECTION('ref_axis',(-0.5,-0.707106781186546,-0.500000000000002));
#27544=DIRECTION('',(0.707106781186548,0.,-0.707106781186548));
#27545=DIRECTION('center_axis',(-0.707106781186548,0.,-0.707106781186548));
#27546=DIRECTION('ref_axis',(0.707106781186548,0.,-0.707106781186548));
#27547=DIRECTION('',(-0.707106781186548,0.,0.707106781186548));
#27548=DIRECTION('center_axis',(0.,-1.,0.));
#27549=DIRECTION('ref_axis',(0.,0.,-1.));
#27550=DIRECTION('center_axis',(0.,-1.,0.));
#27551=DIRECTION('ref_axis',(-0.367874908669274,0.,-0.929875288182008));
#27552=DIRECTION('center_axis',(-0.707106781186548,0.,-0.707106781186547));
#27553=DIRECTION('ref_axis',(-0.499999999999999,-0.707106781186548,0.500000000000001));
#27554=DIRECTION('',(-0.707106781186548,0.,-0.707106781186547));
#27555=DIRECTION('center_axis',(0.,-1.,0.));
#27556=DIRECTION('ref_axis',(0.,0.,-1.));
#27557=DIRECTION('center_axis',(0.,-1.,0.));
#27558=DIRECTION('ref_axis',(-0.899687500253878,0.,-0.436534536877586));
#27559=DIRECTION('center_axis',(0.,-1.,0.));
#27560=DIRECTION('ref_axis',(1.,0.,0.));
#27561=DIRECTION('center_axis',(0.,1.,0.));
#27562=DIRECTION('ref_axis',(1.,0.,0.));
#27563=DIRECTION('',(0.,-1.,0.));
#27564=DIRECTION('center_axis',(-0.707106781186547,0.,0.707106781186548));
#27565=DIRECTION('ref_axis',(-0.707106781186548,0.,-0.707106781186547));
#27566=DIRECTION('',(0.,-1.,0.));
#27567=DIRECTION('',(0.707106781186548,0.,0.707106781186547));
#27568=DIRECTION('center_axis',(0.,-1.,0.));
#27569=DIRECTION('ref_axis',(1.,0.,0.));
#27570=DIRECTION('center_axis',(0.,1.,0.));
#27571=DIRECTION('ref_axis',(1.,0.,0.));
#27572=DIRECTION('center_axis',(0.,1.,0.));
#27573=DIRECTION('ref_axis',(0.,0.,1.));
#27574=DIRECTION('center_axis',(0.,0.,-1.));
#27575=DIRECTION('ref_axis',(0.,1.,0.));
#27576=DIRECTION('center_axis',(1.,0.,0.));
#27577=DIRECTION('ref_axis',(0.,0.,-1.));
#27578=DIRECTION('center_axis',(-1.,0.,0.));
#27579=DIRECTION('ref_axis',(0.,0.707106781186548,-0.707106781186548));
#27580=DIRECTION('center_axis',(1.,0.,-2.96059473233374E-15));
#27581=DIRECTION('ref_axis',(-2.96059473233374E-15,0.,-1.));
#27582=DIRECTION('center_axis',(0.,1.,0.));
#27583=DIRECTION('ref_axis',(0.,0.,1.));
#27584=DIRECTION('center_axis',(0.,0.,-1.));
#27585=DIRECTION('ref_axis',(-1.,0.,0.));
#27586=DIRECTION('center_axis',(0.,0.,1.));
#27587=DIRECTION('ref_axis',(-0.707106781186548,0.707106781186548,0.));
#27588=DIRECTION('center_axis',(-1.48029736616687E-15,0.,-1.));
#27589=DIRECTION('ref_axis',(-1.,0.,1.48029736616687E-15));
#27590=DIRECTION('center_axis',(0.,1.,0.));
#27591=DIRECTION('ref_axis',(0.,0.,1.));
#27592=DIRECTION('center_axis',(-1.,0.,0.));
#27593=DIRECTION('ref_axis',(0.,0.,1.));
#27594=DIRECTION('center_axis',(1.,0.,0.));
#27595=DIRECTION('ref_axis',(0.,0.707106781186548,0.707106781186548));
#27596=DIRECTION('center_axis',(-1.,0.,2.96059473233374E-15));
#27597=DIRECTION('ref_axis',(2.96059473233374E-15,0.,1.));
#27598=DIRECTION('',(1.,0.,0.));
#27599=DIRECTION('center_axis',(0.,1.,0.));
#27600=DIRECTION('ref_axis',(0.,0.,1.));
#27601=DIRECTION('center_axis',(0.,0.,1.));
#27602=DIRECTION('ref_axis',(1.,0.,0.));
#27603=DIRECTION('center_axis',(0.,1.,0.));
#27604=DIRECTION('ref_axis',(0.707106781186547,0.,0.707106781186548));
#27605=DIRECTION('center_axis',(0.,0.,-1.));
#27606=DIRECTION('ref_axis',(0.707106781186548,0.707106781186548,0.));
#27607=DIRECTION('',(0.,0.,-1.));
#27608=DIRECTION('center_axis',(0.,1.,0.));
#27609=DIRECTION('ref_axis',(1.22464679914735E-16,0.,1.));
#27610=DIRECTION('center_axis',(0.,-1.,0.));
#27611=DIRECTION('ref_axis',(1.22464679914735E-16,0.,1.));
#27612=DIRECTION('center_axis',(-1.,0.,-2.46519032881566E-32));
#27613=DIRECTION('ref_axis',(2.46519032881566E-32,0.,-1.));
#27614=DIRECTION('center_axis',(0.,1.,0.));
#27615=DIRECTION('ref_axis',(1.22464679914735E-16,0.,1.));
#27616=DIRECTION('center_axis',(0.,1.,0.));
#27617=DIRECTION('ref_axis',(0.,0.,1.));
#27618=DIRECTION('center_axis',(0.,1.,0.));
#27619=DIRECTION('ref_axis',(0.811029676142761,0.,0.585005012299696));
#27620=DIRECTION('center_axis',(0.,1.,0.));
#27621=DIRECTION('ref_axis',(-0.811029676142761,0.,0.585005012299696));
#27622=DIRECTION('',(0.,-1.,0.));
#27623=DIRECTION('center_axis',(0.,-1.,0.));
#27624=DIRECTION('ref_axis',(0.,0.,-1.));
#27625=DIRECTION('center_axis',(0.,1.,0.));
#27626=DIRECTION('ref_axis',(0.,0.,1.));
#27627=DIRECTION('center_axis',(5.04646829375071E-17,0.,-1.));
#27628=DIRECTION('ref_axis',(-0.707106781186548,-0.707106781186547,0.));
#27629=DIRECTION('',(5.04646829375071E-17,0.,-1.));
#27630=DIRECTION('center_axis',(-1.,0.,-5.04646829375071E-17));
#27631=DIRECTION('ref_axis',(5.04646829375071E-17,0.,-1.));
#27632=DIRECTION('',(-5.04646829375071E-17,0.,1.));
#27633=DIRECTION('center_axis',(0.,1.,0.));
#27634=DIRECTION('ref_axis',(0.,0.,1.));
#27635=DIRECTION('center_axis',(0.,-1.,0.));
#27636=DIRECTION('ref_axis',(0.,0.,-1.));
#27637=DIRECTION('center_axis',(0.,-1.,0.));
#27638=DIRECTION('ref_axis',(0.811029676142761,0.,0.585005012299696));
#27639=DIRECTION('center_axis',(0.,1.,0.));
#27640=DIRECTION('ref_axis',(1.,0.,0.));
#27641=DIRECTION('center_axis',(0.,1.,0.));
#27642=DIRECTION('ref_axis',(0.,0.,1.));
#27643=DIRECTION('center_axis',(0.,-1.,0.));
#27644=DIRECTION('ref_axis',(0.,0.,-1.));
#27645=DIRECTION('center_axis',(0.,-1.,0.));
#27646=DIRECTION('ref_axis',(-0.811029676142761,0.,0.585005012299696));
#27647=DIRECTION('center_axis',(0.,1.,0.));
#27648=DIRECTION('ref_axis',(1.,0.,0.));
#27649=DIRECTION('center_axis',(0.,0.,1.));
#27650=DIRECTION('ref_axis',(-0.707106781186545,0.70710678118655,0.));
#27651=DIRECTION('center_axis',(0.,0.,1.));
#27652=DIRECTION('ref_axis',(0.,1.,0.));
#27653=DIRECTION('',(0.,0.,1.));
#27654=DIRECTION('center_axis',(9.5625613772925E-16,0.,-1.));
#27655=DIRECTION('ref_axis',(-1.,0.,-9.5625613772925E-16));
#27656=DIRECTION('center_axis',(0.,-1.,0.));
#27657=DIRECTION('ref_axis',(-1.22464679914735E-16,0.,1.));
#27658=DIRECTION('center_axis',(0.,0.,1.));
#27659=DIRECTION('ref_axis',(1.,0.,0.));
#27660=DIRECTION('center_axis',(0.,-1.,0.));
#27661=DIRECTION('ref_axis',(-6.12323399573677E-17,0.,1.));
#27662=DIRECTION('center_axis',(0.,0.,-1.));
#27663=DIRECTION('ref_axis',(0.707106781186545,0.70710678118655,0.));
#27664=DIRECTION('center_axis',(0.,0.,1.));
#27665=DIRECTION('ref_axis',(1.,0.,0.));
#27666=DIRECTION('',(0.,0.,-1.));
#27667=DIRECTION('center_axis',(0.,-1.,0.));
#27668=DIRECTION('ref_axis',(0.,0.,-1.));
#27669=DIRECTION('center_axis',(0.,-1.,0.));
#27670=DIRECTION('ref_axis',(6.12323399573677E-17,0.,-1.));
#27671=DIRECTION('center_axis',(0.,-1.,0.));
#27672=DIRECTION('ref_axis',(-1.,0.,0.));
#27673=DIRECTION('',(0.,-1.,0.));
#27674=DIRECTION('center_axis',(0.,-1.,0.));
#27675=DIRECTION('ref_axis',(-1.,0.,0.));
#27676=DIRECTION('',(0.,-1.,0.));
#27677=DIRECTION('center_axis',(1.,0.,0.));
#27678=DIRECTION('ref_axis',(0.,0.,1.));
#27679=DIRECTION('',(0.,-1.,0.));
#27680=DIRECTION('',(0.,0.,1.));
#27681=DIRECTION('center_axis',(0.,0.,1.));
#27682=DIRECTION('ref_axis',(-0.707106781186545,0.70710678118655,0.));
#27683=DIRECTION('center_axis',(0.,0.,1.));
#27684=DIRECTION('ref_axis',(0.,1.,0.));
#27685=DIRECTION('',(0.,0.,1.));
#27686=DIRECTION('center_axis',(0.,0.,-1.));
#27687=DIRECTION('ref_axis',(-1.,0.,0.));
#27688=DIRECTION('center_axis',(0.,1.,0.));
#27689=DIRECTION('ref_axis',(0.,0.,1.));
#27690=DIRECTION('center_axis',(-1.22464679914735E-16,0.,1.));
#27691=DIRECTION('ref_axis',(1.,0.,1.22464679914735E-16));
#27692=DIRECTION('center_axis',(0.,1.,0.));
#27693=DIRECTION('ref_axis',(-6.12323399573676E-17,0.,1.));
#27694=DIRECTION('center_axis',(0.,0.,-1.));
#27695=DIRECTION('ref_axis',(0.707106781186545,0.70710678118655,0.));
#27696=DIRECTION('center_axis',(0.,0.,1.));
#27697=DIRECTION('ref_axis',(1.,0.,0.));
#27698=DIRECTION('',(0.,0.,-1.));
#27699=DIRECTION('center_axis',(0.,1.,0.));
#27700=DIRECTION('ref_axis',(-1.22464679914735E-16,0.,-1.));
#27701=DIRECTION('center_axis',(0.,1.,0.));
#27702=DIRECTION('ref_axis',(8.54643792476272E-17,0.,-1.));
#27703=DIRECTION('center_axis',(0.,-1.,0.));
#27704=DIRECTION('ref_axis',(-1.,0.,0.));
#27705=DIRECTION('',(0.,-1.,0.));
#27706=DIRECTION('center_axis',(0.,1.,0.));
#27707=DIRECTION('ref_axis',(-1.,0.,0.));
#27708=DIRECTION('',(0.,-1.,0.));
#27709=DIRECTION('center_axis',(1.,0.,0.));
#27710=DIRECTION('ref_axis',(0.,0.,1.));
#27711=DIRECTION('',(0.,-1.,0.));
#27712=DIRECTION('',(0.,0.,1.));
#27713=DIRECTION('center_axis',(0.,-1.,0.));
#27714=DIRECTION('ref_axis',(1.,0.,-1.97812565634772E-16));
#27715=DIRECTION('',(0.,-1.,0.));
#27716=DIRECTION('center_axis',(0.,1.,0.));
#27717=DIRECTION('ref_axis',(1.,0.,-1.97812565634772E-16));
#27718=DIRECTION('center_axis',(-1.,0.,0.));
#27719=DIRECTION('ref_axis',(0.,0.,-1.));
#27720=DIRECTION('',(0.,0.,-1.));
#27721=DIRECTION('center_axis',(0.,-1.,0.));
#27722=DIRECTION('ref_axis',(1.,0.,0.));
#27723=DIRECTION('',(0.,-1.,0.));
#27724=DIRECTION('center_axis',(0.,-1.,0.));
#27725=DIRECTION('ref_axis',(1.,0.,0.));
#27726=DIRECTION('center_axis',(-1.,0.,0.));
#27727=DIRECTION('ref_axis',(0.,0.,-1.));
#27728=DIRECTION('',(0.,0.,-1.));
#27729=DIRECTION('center_axis',(0.,1.,0.));
#27730=DIRECTION('ref_axis',(1.,0.,0.));
#27731=DIRECTION('center_axis',(0.,-1.,0.));
#27732=DIRECTION('ref_axis',(1.,0.,0.));
#27733=DIRECTION('',(0.,-1.,0.));
#27734=DIRECTION('center_axis',(0.,-1.,0.));
#27735=DIRECTION('ref_axis',(1.,0.,0.));
#27736=DIRECTION('center_axis',(0.,1.,0.));
#27737=DIRECTION('ref_axis',(1.,0.,0.));
#27738=DIRECTION('center_axis',(0.,-1.,0.));
#27739=DIRECTION('ref_axis',(1.,0.,0.));
#27740=DIRECTION('',(0.,-1.,0.));
#27741=DIRECTION('center_axis',(0.,-1.,0.));
#27742=DIRECTION('ref_axis',(1.,0.,0.));
#27743=DIRECTION('center_axis',(0.,1.,0.));
#27744=DIRECTION('ref_axis',(1.,0.,0.));
#27745=DIRECTION('center_axis',(0.,-1.,0.));
#27746=DIRECTION('ref_axis',(0.,0.,-1.));
#27747=DIRECTION('center_axis',(0.,1.,0.));
#27748=DIRECTION('ref_axis',(1.,0.,0.));
#27749=DIRECTION('center_axis',(0.,1.,0.));
#27750=DIRECTION('ref_axis',(0.,0.,1.));
#27751=DIRECTION('center_axis',(0.,1.,0.));
#27752=DIRECTION('ref_axis',(0.,0.,1.));
#27753=DIRECTION('',(0.,1.,0.));
#27754=DIRECTION('center_axis',(0.,1.,0.));
#27755=DIRECTION('ref_axis',(1.,0.,0.));
#27756=DIRECTION('center_axis',(0.,1.,0.));
#27757=DIRECTION('ref_axis',(0.,0.,1.));
#27758=DIRECTION('center_axis',(0.,-1.,0.));
#27759=DIRECTION('ref_axis',(0.,0.,1.));
#27760=DIRECTION('center_axis',(0.,1.,0.));
#27761=DIRECTION('ref_axis',(0.,0.,1.));
#27762=DIRECTION('',(0.,1.,0.));
#27763=DIRECTION('center_axis',(0.,1.,0.));
#27764=DIRECTION('ref_axis',(0.,0.,1.));
#27765=DIRECTION('',(0.,1.,0.));
#27766=DIRECTION('center_axis',(0.,1.,0.));
#27767=DIRECTION('ref_axis',(1.,0.,0.));
#27768=DIRECTION('center_axis',(0.,-1.,0.));
#27769=DIRECTION('ref_axis',(1.,0.,0.));
#27770=DIRECTION('center_axis',(0.,1.,0.));
#27771=DIRECTION('ref_axis',(1.,0.,0.));
#27772=DIRECTION('',(0.,1.,0.));
#27773=DIRECTION('center_axis',(0.,-1.,0.));
#27774=DIRECTION('ref_axis',(1.,0.,0.));
#27775=DIRECTION('center_axis',(0.,1.,0.));
#27776=DIRECTION('ref_axis',(1.,0.,0.));
#27777=DIRECTION('',(0.,1.,0.));
#27778=DIRECTION('center_axis',(0.,1.,0.));
#27779=DIRECTION('ref_axis',(1.,0.,0.));
#27780=DIRECTION('',(1.,0.,0.));
#27781=DIRECTION('center_axis',(0.,0.,1.));
#27782=DIRECTION('ref_axis',(1.,0.,0.));
#27783=DIRECTION('',(0.,1.,0.));
#27784=DIRECTION('center_axis',(-1.,0.,0.));
#27785=DIRECTION('ref_axis',(0.,0.,1.));
#27786=DIRECTION('',(0.,0.,1.));
#27787=DIRECTION('center_axis',(0.,0.,1.));
#27788=DIRECTION('ref_axis',(1.,0.,0.));
#27789=DIRECTION('',(1.,0.,0.));
#27790=DIRECTION('center_axis',(0.,1.,0.));
#27791=DIRECTION('ref_axis',(1.,0.,0.));
#27792=DIRECTION('center_axis',(0.,1.,0.));
#27793=DIRECTION('ref_axis',(1.,0.,0.));
#27794=DIRECTION('center_axis',(1.,0.,0.));
#27795=DIRECTION('ref_axis',(0.,0.,-1.));
#27796=DIRECTION('',(0.,1.,0.));
#27797=DIRECTION('center_axis',(0.,1.,0.));
#27798=DIRECTION('ref_axis',(4.75809867696496E-16,0.,1.));
#33457=CARTESIAN_POINT('',(0.,0.,0.));
#33458=CARTESIAN_POINT('Origin',(30.5,0.25,-55.));
#33459=CARTESIAN_POINT('',(22.,0.,-55.));
#33460=CARTESIAN_POINT('Origin',(30.5,0.,-55.));
#33461=CARTESIAN_POINT('',(21.5,0.5,-55.));
#33462=CARTESIAN_POINT('',(21.75,0.25,-55.));
#33463=CARTESIAN_POINT('Origin',(30.5,0.5,-55.));
#33464=CARTESIAN_POINT('Origin',(30.5,0.,-55.));
#33465=CARTESIAN_POINT('',(24.95,0.,-55.));
#33466=CARTESIAN_POINT('Origin',(30.5,0.,-55.));
#33467=CARTESIAN_POINT('Origin',(30.5,4.,-55.));
#33468=CARTESIAN_POINT('',(21.5,4.,-55.));
#33469=CARTESIAN_POINT('',(21.5,4.,-55.));
#33470=CARTESIAN_POINT('Origin',(30.5,4.,-55.));
#33471=CARTESIAN_POINT('Origin',(-30.5,0.25,-55.));
#33472=CARTESIAN_POINT('',(-39.,0.,-55.));
#33473=CARTESIAN_POINT('Origin',(-30.5,0.,-55.));
#33474=CARTESIAN_POINT('',(-39.5,0.5,-55.));
#33475=CARTESIAN_POINT('',(-39.25,0.25,-55.));
#33476=CARTESIAN_POINT('Origin',(-30.5,0.5,-55.));
#33477=CARTESIAN_POINT('Origin',(-30.5,0.,-55.));
#33478=CARTESIAN_POINT('',(-36.05,0.,-55.));
#33479=CARTESIAN_POINT('Origin',(-30.5,0.,-55.));
#33480=CARTESIAN_POINT('Origin',(-30.5,4.,-55.));
#33481=CARTESIAN_POINT('',(-39.5,4.,-55.));
#33482=CARTESIAN_POINT('',(-39.5,4.,-55.));
#33483=CARTESIAN_POINT('Origin',(-30.5,4.,-55.));
#33484=CARTESIAN_POINT('Origin',(0.,2.35,0.));
#33485=CARTESIAN_POINT('',(-1.28587913910472E-15,2.1,10.5));
#33486=CARTESIAN_POINT('Origin',(0.,2.1,0.));
#33487=CARTESIAN_POINT('',(1.22464679914735E-15,2.6,10.));
#33488=CARTESIAN_POINT('',(-1.25526296912604E-15,2.35,10.25));
#33489=CARTESIAN_POINT('',(-1.22464679914735E-15,2.6,-10.));
#33490=CARTESIAN_POINT('Origin',(0.,2.6,0.));
#33491=CARTESIAN_POINT('Origin',(0.,2.6,0.));
#33492=CARTESIAN_POINT('Origin',(0.,10.1,0.));
#33493=CARTESIAN_POINT('',(1.22464679914735E-15,17.5,-10.));
#33494=CARTESIAN_POINT('',(-1.22464679914735E-15,10.1,-10.));
#33495=CARTESIAN_POINT('Origin',(0.,17.5,0.));
#33496=CARTESIAN_POINT('Origin',(0.,2.1,10.));
#33497=CARTESIAN_POINT('',(-1.75124492278072E-15,2.1,-14.3));
#33498=CARTESIAN_POINT('Origin',(0.,2.1,0.));
#33499=CARTESIAN_POINT('Origin',(0.,17.75,0.));
#33500=CARTESIAN_POINT('',(-1.28587913910472E-15,18.,-10.5));
#33501=CARTESIAN_POINT('Origin',(0.,18.,0.));
#33502=CARTESIAN_POINT('',(-1.25526296912604E-15,17.75,-10.25));
#33503=CARTESIAN_POINT('Origin',(0.,18.,-16.5));
#33504=CARTESIAN_POINT('',(-20.95,18.,0.));
#33505=CARTESIAN_POINT('',(-20.95,18.,-33.));
#33506=CARTESIAN_POINT('',(-20.95,18.,-24.75));
#33507=CARTESIAN_POINT('',(20.95,18.,2.5656350442137E-15));
#33508=CARTESIAN_POINT('Origin',(0.,18.,0.));
#33509=CARTESIAN_POINT('',(20.95,18.,-33.));
#33510=CARTESIAN_POINT('',(20.95,18.,-8.25));
#33511=CARTESIAN_POINT('Origin',(0.,18.,-33.));
#33512=CARTESIAN_POINT('Ctrl Pts',(-1.57453458878625,0.00185294611160958,
-63.8682453580158));
#33513=CARTESIAN_POINT('Ctrl Pts',(-1.57038661518133,0.00164657951619636,
-63.8641633585059));
#33514=CARTESIAN_POINT('Ctrl Pts',(-1.539887259118,0.000219540540016254,
-63.8342603933394));
#33515=CARTESIAN_POINT('Ctrl Pts',(-1.50642463475971,1.28888202266086E-5,
-63.8016081711826));
#33516=CARTESIAN_POINT('Ctrl Pts',(-1.50104102377551,-5.7788428237887E-19,
-63.7963365978802));
#33517=CARTESIAN_POINT('Ctrl Pts',(-1.5,0.,-63.7953186364093));
#33518=CARTESIAN_POINT('Ctrl Pts',(-1.3391048451961,0.00185294611160958,
-64.1036751016059));
#33519=CARTESIAN_POINT('Ctrl Pts',(-1.3349788629562,0.00164657951619632,
-64.0995711107311));
#33520=CARTESIAN_POINT('Ctrl Pts',(-1.30471094646532,0.000219540540016221,
-64.0694367059921));
#33521=CARTESIAN_POINT('Ctrl Pts',(-1.27147622898836,1.2888820226605E-5,
-64.0365565769539));
#33522=CARTESIAN_POINT('Ctrl Pts',(-1.26613954847708,-3.55392112035979E-19,
-64.0312380731786));
#33523=CARTESIAN_POINT('Ctrl Pts',(-1.26510621213642,0.,-64.0302124242728));
#33524=CARTESIAN_POINT('Ctrl Pts',(-1.10367510160594,0.00185294611160958,
-64.3391048451961));
#33525=CARTESIAN_POINT('Ctrl Pts',(-1.09957111073107,0.00164657951619628,
-64.3349788629562));
#33526=CARTESIAN_POINT('Ctrl Pts',(-1.0694367059921,-2.15946827128807E-5,
-64.3045339520233));
#33527=CARTESIAN_POINT('Ctrl Pts',(-1.0365565769539,0.000165305522380892,
-64.2714516442099));
#33528=CARTESIAN_POINT('Ctrl Pts',(-1.03123807317865,-1.23401226123361E-19,
-64.2661395484771));
#33529=CARTESIAN_POINT('Ctrl Pts',(-1.03021242427284,0.,-64.2651062121364));
#33530=CARTESIAN_POINT('Ctrl Pts',(-0.868245358015784,0.00185294611160958,
-64.5745345887862));
#33531=CARTESIAN_POINT('Ctrl Pts',(-0.864163358505944,0.00164657951619624,
-64.5703866151813));
#33532=CARTESIAN_POINT('Ctrl Pts',(-0.834260393339416,0.000219540540015427,
-64.539887259118));
#33533=CARTESIAN_POINT('Ctrl Pts',(-0.801608171182549,1.28888202263444E-5,
-64.5064246347597));
#33534=CARTESIAN_POINT('Ctrl Pts',(-0.796336597880214,9.63140470631229E-20,
-64.5010410237755));
#33535=CARTESIAN_POINT('Ctrl Pts',(-0.79531863640926,0.,-64.5));
#33536=CARTESIAN_POINT('',(-1.5,0.,-63.7953186364093));
#33537=CARTESIAN_POINT('',(-1.57453458878625,0.00185294611160958,-63.8682453580158));
#33538=CARTESIAN_POINT('Ctrl Pts',(-1.49999999999999,-2.22044604925031E-16,
-63.7953186364093));
#33539=CARTESIAN_POINT('Ctrl Pts',(-1.50033136103367,-2.2224081007119E-16,
-63.7956426566413));
#33540=CARTESIAN_POINT('Ctrl Pts',(-1.50066599103948,9.12216844759869E-8,
-63.7959698710105));
#33541=CARTESIAN_POINT('Ctrl Pts',(-1.50107815475909,3.87472611551587E-7,
-63.7963728195339));
#33542=CARTESIAN_POINT('Ctrl Pts',(-1.50151072778695,6.98393137628669E-7,
-63.7967957210522));
#33543=CARTESIAN_POINT('Ctrl Pts',(-1.5020284953742,1.23194503946057E-6,
-63.7973018394014));
#33544=CARTESIAN_POINT('Ctrl Pts',(-1.50267576544792,2.38657547568799E-6,
-63.7979344421873));
#33545=CARTESIAN_POINT('Ctrl Pts',(-1.50336536547683,3.6167160530659E-6,
-63.798608415722));
#33546=CARTESIAN_POINT('Ctrl Pts',(-1.50420167541466,5.55516755071447E-6,
-63.7994256794685));
#33547=CARTESIAN_POINT('Ctrl Pts',(-1.50519595537272,8.99934440767858E-6,
-63.8003972134394));
#33548=CARTESIAN_POINT('Ctrl Pts',(-1.50629355744866,1.28014281542221E-5,
-63.8014697058442));
#33549=CARTESIAN_POINT('Ctrl Pts',(-1.50758325228905,1.84658046861493E-5,
-63.802729790879));
#33550=CARTESIAN_POINT('Ctrl Pts',(-1.50903534240277,2.72127176224046E-5,
-63.8041484437088));
#33551=CARTESIAN_POINT('Ctrl Pts',(-1.51085714423942,3.81866522988828E-5,
-63.8059282949085));
#33552=CARTESIAN_POINT('Ctrl Pts',(-1.51293366154185,5.41281456159546E-5,
-63.8079568545962));
#33553=CARTESIAN_POINT('Ctrl Pts',(-1.5151467124789,7.64762491785032E-5,
-63.8101187023241));
#33554=CARTESIAN_POINT('Ctrl Pts',(-1.51749449195499,0.000100184885069023,
-63.812412161386));
#33555=CARTESIAN_POINT('Ctrl Pts',(-1.51999108760992,0.000131146817808081,
-63.8148508937682));
#33556=CARTESIAN_POINT('Ctrl Pts',(-1.52248486630875,0.000168532538713073,
-63.8172869062401));
#33557=CARTESIAN_POINT('Ctrl Pts',(-1.52437422457671,0.000196857033155279,
-63.8191324991577));
#33558=CARTESIAN_POINT('Ctrl Pts',(-1.52626114404841,0.000228767928628635,
-63.8209757293306));
#33559=CARTESIAN_POINT('Ctrl Pts',(-1.52810370841056,0.000263295917055206,
-63.8227757579307));
#33560=CARTESIAN_POINT('Ctrl Pts',(-1.5297663700739,0.000294452691737526,
-63.8244000369018));
#33561=CARTESIAN_POINT('Ctrl Pts',(-1.53139250445785,0.000327690884682965,
-63.8259887368552));
#33562=CARTESIAN_POINT('Ctrl Pts',(-1.53298085050773,0.00036262266513698,
-63.8275407505537));
#33563=CARTESIAN_POINT('Ctrl Pts',(-1.53454774391469,0.000397082647261587,
-63.829071802324));
#33564=CARTESIAN_POINT('Ctrl Pts',(-1.53607719242315,0.000433137034783167,
-63.8305664957212));
#33565=CARTESIAN_POINT('Ctrl Pts',(-1.53760652085703,0.000471490904881078,
-63.8320614739056));
#33566=CARTESIAN_POINT('Ctrl Pts',(-1.53909804395478,0.000508896658852536,
-63.8335194958996));
#33567=CARTESIAN_POINT('Ctrl Pts',(-1.5405961355825,0.000548663598858774,
-63.8349843334466));
#33568=CARTESIAN_POINT('Ctrl Pts',(-1.54213060631517,0.000591779397113079,
-63.8364852326094));
#33569=CARTESIAN_POINT('Ctrl Pts',(-1.54377985735777,0.000638120310438484,
-63.838098400887));
#33570=CARTESIAN_POINT('Ctrl Pts',(-1.54547077478746,0.000688360290152192,
-63.8397528770161));
#33571=CARTESIAN_POINT('Ctrl Pts',(-1.54719744053054,0.000742716673563626,
-63.8414428847976));
#33572=CARTESIAN_POINT('Ctrl Pts',(-1.54917002631339,0.00080481475453534,
-63.8433735916157));
#33573=CARTESIAN_POINT('Ctrl Pts',(-1.55118873161025,0.000872336312443033,
-63.8453501484937));
#33574=CARTESIAN_POINT('Ctrl Pts',(-1.55319701397665,0.000943604228323958,
-63.8473171286807));
#33575=CARTESIAN_POINT('Ctrl Pts',(-1.55597939118099,0.00104234244754321,
-63.8500422837313));
#33576=CARTESIAN_POINT('Ctrl Pts',(-1.55873880451989,0.00114840209592754,
-63.8527461713318));
#33577=CARTESIAN_POINT('Ctrl Pts',(-1.56125854441685,0.00125139174845978,
-63.8552161386877));
#33578=CARTESIAN_POINT('Ctrl Pts',(-1.56314834933957,0.00132863398785897,
-63.8570686142046));
#33579=CARTESIAN_POINT('Ctrl Pts',(-1.56490064570691,0.00140389724196252,
-63.8587868623066));
#33580=CARTESIAN_POINT('Ctrl Pts',(-1.56643959313722,0.00147212889991266,
-63.8602963585415));
#33581=CARTESIAN_POINT('Ctrl Pts',(-1.5677289530965,0.00152929470426916,
-63.8615610437189));
#33582=CARTESIAN_POINT('Ctrl Pts',(-1.568868184354,0.00158146111032055,
-63.8626788313975));
#33583=CARTESIAN_POINT('Ctrl Pts',(-1.56983898661494,0.0016267100790277,
-63.8636316653217));
#33584=CARTESIAN_POINT('Ctrl Pts',(-1.57075171477114,0.00166925222117146,
-63.8645275000202));
#33585=CARTESIAN_POINT('Ctrl Pts',(-1.571515145023,0.00170564250684221,
-63.8652771155594));
#33586=CARTESIAN_POINT('Ctrl Pts',(-1.57214502087141,0.00173597254573887,
-63.8658958651526));
#33587=CARTESIAN_POINT('Ctrl Pts',(-1.57273209133851,0.00176424140244595,
-63.8664725654875));
#33588=CARTESIAN_POINT('Ctrl Pts',(-1.57320299278075,0.00178723762245352,
-63.8669354348749));
#33589=CARTESIAN_POINT('Ctrl Pts',(-1.57360188999628,0.00180683428705497,
-63.867327729259));
#33590=CARTESIAN_POINT('Ctrl Pts',(-1.57394979081276,0.00182392564630744,
-63.8676698713729));
#33591=CARTESIAN_POINT('Ctrl Pts',(-1.57424318974083,0.0018384486642682,
-63.8679585937126));
#33592=CARTESIAN_POINT('Ctrl Pts',(-1.57453458878625,0.00185294611160969,
-63.8682453580158));
#33593=CARTESIAN_POINT('',(-0.868245358015784,0.00185294611160958,-64.5745345887862));
#33594=CARTESIAN_POINT('Ctrl Pts',(-0.868245358015784,0.00185294611160958,
-64.5745345887862));
#33595=CARTESIAN_POINT('Ctrl Pts',(-1.10367510160594,0.00185294611160958,
-64.3391048451961));
#33596=CARTESIAN_POINT('Ctrl Pts',(-1.3391048451961,0.00185294611160958,
-64.1036751016059));
#33597=CARTESIAN_POINT('Ctrl Pts',(-1.57453458878625,0.00185294611160958,
-63.8682453580158));
#33598=CARTESIAN_POINT('',(-0.79531863640926,0.,-64.5));
#33599=CARTESIAN_POINT('Ctrl Pts',(-0.868245358015784,0.00185294611160947,
-64.5745345887863));
#33600=CARTESIAN_POINT('Ctrl Pts',(-0.867920511984305,0.00183652343213872,
-64.5742044925281));
#33601=CARTESIAN_POINT('Ctrl Pts',(-0.867592467561066,0.00182002913551296,
-64.5738711310018));
#33602=CARTESIAN_POINT('Ctrl Pts',(-0.867188603524973,0.00179989061882035,
-64.57346041281));
#33603=CARTESIAN_POINT('Ctrl Pts',(-0.866764739391085,0.00177875480534643,
-64.57302935509));
#33604=CARTESIAN_POINT('Ctrl Pts',(-0.86625756382414,0.00175361200744126,
-64.5725132968389));
#33605=CARTESIAN_POINT('Ctrl Pts',(-0.865623769120512,0.00172265954511208,
-64.5718680115171));
#33606=CARTESIAN_POINT('Ctrl Pts',(-0.864948520897705,0.00168968262836025,
-64.5711805211291));
#33607=CARTESIAN_POINT('Ctrl Pts',(-0.864129827824869,0.00165012867729293,
-64.5703466306137));
#33608=CARTESIAN_POINT('Ctrl Pts',(-0.86315671761943,0.001604232339808,
-64.5693550535868));
#33609=CARTESIAN_POINT('Ctrl Pts',(-0.862082460752306,0.00155356546215793,
-64.5682604104266));
#33610=CARTESIAN_POINT('Ctrl Pts',(-0.860820424065946,0.00149521701853039,
-64.5669740091159));
#33611=CARTESIAN_POINT('Ctrl Pts',(-0.859399706742866,0.00143187557828406,
-64.565525387959));
#33612=CARTESIAN_POINT('Ctrl Pts',(-0.857617058277222,0.00135239775434793,
-64.5637077270911));
#33613=CARTESIAN_POINT('Ctrl Pts',(-0.855585466407158,0.00126521876821512,
-64.5616355608823));
#33614=CARTESIAN_POINT('Ctrl Pts',(-0.853420628947171,0.00117763891592859,
-64.5594266767906));
#33615=CARTESIAN_POINT('Ctrl Pts',(-0.851124884258546,0.00108476312990145,
-64.5570842219804));
#33616=CARTESIAN_POINT('Ctrl Pts',(-0.848684033523705,0.000991719524374041,
-64.5545928471898));
#33617=CARTESIAN_POINT('Ctrl Pts',(-0.846246251751938,0.00090520107638592,
-64.552103587594));
#33618=CARTESIAN_POINT('Ctrl Pts',(-0.844398979277231,0.000839640184359459,
-64.5502173068831));
#33619=CARTESIAN_POINT('Ctrl Pts',(-0.842554271958467,0.000777766532134859,
-64.5483330647398));
#33620=CARTESIAN_POINT('Ctrl Pts',(-0.840753063942645,0.000720694561445301,
-64.5464926261216));
#33621=CARTESIAN_POINT('Ctrl Pts',(-0.839127695829264,0.000669194145884327,
-64.5448318572274));
#33622=CARTESIAN_POINT('Ctrl Pts',(-0.837538150811472,0.000621574660655034,
-64.543207168852));
#33623=CARTESIAN_POINT('Ctrl Pts',(-0.835985578644532,0.000577512604326147,
-64.5416197584348));
#33624=CARTESIAN_POINT('Ctrl Pts',(-0.83445351746975,0.00053403265072395,
-64.540053319257));
#33625=CARTESIAN_POINT('Ctrl Pts',(-0.832958118217025,0.000493996445435221,
-64.5385238533706));
#33626=CARTESIAN_POINT('Ctrl Pts',(-0.831462700584247,0.000456253937660245,
-64.5369939676883));
#33627=CARTESIAN_POINT('Ctrl Pts',(-0.830004714201859,0.000419456148757018,
-64.5355023760136));
#33628=CARTESIAN_POINT('Ctrl Pts',(-0.828540166631002,0.000384680303812991,
-64.5340037037557));
#33629=CARTESIAN_POINT('Ctrl Pts',(-0.827039815786342,0.000351435419327029,
-64.5324681805947));
#33630=CARTESIAN_POINT('Ctrl Pts',(-0.825427211040693,0.000315703204637751,
-64.530817771995));
#33631=CARTESIAN_POINT('Ctrl Pts',(-0.823773595132572,0.000281787957708217,
-64.529125149268));
#33632=CARTESIAN_POINT('Ctrl Pts',(-0.822084705002914,0.000250206967384647,
-64.5273963190708));
#33633=CARTESIAN_POINT('Ctrl Pts',(-0.820155155817438,0.00021412583156339,
-64.5254211385423));
#33634=CARTESIAN_POINT('Ctrl Pts',(-0.818180086158876,0.000181169469766856,
-64.5233992312895));
#33635=CARTESIAN_POINT('Ctrl Pts',(-0.816214827518119,0.000152480845410752,
-64.5213873627599));
#33636=CARTESIAN_POINT('Ctrl Pts',(-0.813492568573185,0.000112741615850007,
-64.5186005402078));
#33637=CARTESIAN_POINT('Ctrl Pts',(-0.810792018065188,8.14691463192202E-5,
-64.5158359360067));
#33638=CARTESIAN_POINT('Ctrl Pts',(-0.808325391140352,5.90616066569183E-5,
-64.5133109478137));
#33639=CARTESIAN_POINT('Ctrl Pts',(-0.806475420946726,4.22559519101918E-5,
-64.5114172066688));
#33640=CARTESIAN_POINT('Ctrl Pts',(-0.804759675671119,3.03183594525773E-5,
-64.5096609508553));
#33641=CARTESIAN_POINT('Ctrl Pts',(-0.803252515255964,2.19691435532354E-5,
-64.5081183094309));
#33642=CARTESIAN_POINT('Ctrl Pts',(-0.801989757154794,1.49738430468668E-5,
-64.5068258239488));
#33643=CARTESIAN_POINT('Ctrl Pts',(-0.800873785775093,1.04521897691688E-5,
-64.5056836631396));
#33644=CARTESIAN_POINT('Ctrl Pts',(-0.799922600320211,7.39546431272053E-6,
-64.5047102375997));
#33645=CARTESIAN_POINT('Ctrl Pts',(-0.799028303767072,4.52155678442164E-6,
-64.5037950311059));
#33646=CARTESIAN_POINT('Ctrl Pts',(-0.798280081319924,2.92603171309864E-6,
-64.5030293988184));
#33647=CARTESIAN_POINT('Ctrl Pts',(-0.797662574868972,1.91616332645417E-6,
-64.5023976001144));
#33648=CARTESIAN_POINT('Ctrl Pts',(-0.797087026101143,9.74912421775467E-7,
-64.5018087302087));
#33649=CARTESIAN_POINT('Ctrl Pts',(-0.796625180682792,5.41797940511647E-7,
-64.5013362750361));
#33650=CARTESIAN_POINT('Ctrl Pts',(-0.796233819415205,2.9201856199812E-7,
-64.500935978419));
#33651=CARTESIAN_POINT('Ctrl Pts',(-0.795892553137518,7.42114211081106E-8,
-64.5005869205336));
#33652=CARTESIAN_POINT('Ctrl Pts',(-0.795604617783312,-2.22022958507712E-16,
-64.5002924603909));
#33653=CARTESIAN_POINT('Ctrl Pts',(-0.79531863640926,-2.22044604925031E-16,
-64.5));
#33654=CARTESIAN_POINT('',(-1.14765931820463,0.,-64.1476593182046));
#33655=CARTESIAN_POINT('Ctrl Pts',(-0.868245358015784,0.00185294611160958,
-64.5745345887862));
#33656=CARTESIAN_POINT('Ctrl Pts',(-1.24643975969902,0.0209726669473527,
-64.9588414442702));
#33657=CARTESIAN_POINT('Ctrl Pts',(-1.89279714334289,0.308835349231178,
-65.5507400778319));
#33658=CARTESIAN_POINT('Ctrl Pts',(-2.42122743991223,0.985650418224739,
-65.9509027104217));
#33659=CARTESIAN_POINT('Ctrl Pts',(-2.49999999999999,1.33275179473161,-66.));
#33660=CARTESIAN_POINT('Ctrl Pts',(-2.49999999999999,1.5,-66.));
#33661=CARTESIAN_POINT('Ctrl Pts',(-1.10367510160594,0.00185294611160958,
-64.3391048451961));
#33662=CARTESIAN_POINT('Ctrl Pts',(-1.48390698788943,0.020972666947353,
-64.7213742160798));
#33663=CARTESIAN_POINT('Ctrl Pts',(-2.11211145483922,0.308835349231178,
-65.3314257663356));
#33664=CARTESIAN_POINT('Ctrl Pts',(-2.59778586341538,0.985650418224741,
-65.7743442869185));
#33665=CARTESIAN_POINT('Ctrl Pts',(-2.66666666666666,1.33275179473161,-65.8333333333333));
#33666=CARTESIAN_POINT('Ctrl Pts',(-2.66666666666666,1.5,-65.8333333333333));
#33667=CARTESIAN_POINT('Ctrl Pts',(-1.3391048451961,0.00185294611160958,
-64.1036751016059));
#33668=CARTESIAN_POINT('Ctrl Pts',(-1.72137421607983,0.0209726669473534,
-64.4839069878894));
#33669=CARTESIAN_POINT('Ctrl Pts',(-2.33142576633555,0.308835349231176,
-65.1121114548392));
#33670=CARTESIAN_POINT('Ctrl Pts',(-2.77434428691853,0.985650418224743,
-65.5977858634154));
#33671=CARTESIAN_POINT('Ctrl Pts',(-2.83333333333333,1.33275179473161,-65.6666666666667));
#33672=CARTESIAN_POINT('Ctrl Pts',(-2.83333333333333,1.5,-65.6666666666667));
#33673=CARTESIAN_POINT('Ctrl Pts',(-1.57453458878625,0.00185294611160958,
-63.8682453580158));
#33674=CARTESIAN_POINT('Ctrl Pts',(-1.95884144427023,0.0209726669473537,
-64.246439759699));
#33675=CARTESIAN_POINT('Ctrl Pts',(-2.55074007783188,0.308835349231176,
-64.8927971433429));
#33676=CARTESIAN_POINT('Ctrl Pts',(-2.95090271042168,0.985650418224745,
-65.4212274399123));
#33677=CARTESIAN_POINT('Ctrl Pts',(-3.,1.33275179473161,-65.5));
#33678=CARTESIAN_POINT('Ctrl Pts',(-3.,1.5,-65.5));
#33679=CARTESIAN_POINT('',(-3.,1.5,-65.5));
#33680=CARTESIAN_POINT('Ctrl Pts',(-1.57453458878625,0.00185294611160958,
-63.8682453580158));
#33681=CARTESIAN_POINT('Ctrl Pts',(-1.95884144427023,0.0209726669473537,
-64.246439759699));
#33682=CARTESIAN_POINT('Ctrl Pts',(-2.55074007783188,0.308835349231176,
-64.8927971433429));
#33683=CARTESIAN_POINT('Ctrl Pts',(-2.95090271042168,0.985650418224745,
-65.4212274399123));
#33684=CARTESIAN_POINT('Ctrl Pts',(-3.,1.33275179473161,-65.5));
#33685=CARTESIAN_POINT('Ctrl Pts',(-3.,1.5,-65.5));
#33686=CARTESIAN_POINT('',(-2.49999999999999,1.5,-66.));
#33687=CARTESIAN_POINT('',(-3.,1.5,-65.5));
#33688=CARTESIAN_POINT('Ctrl Pts',(-2.49999999999999,1.5,-66.));
#33689=CARTESIAN_POINT('Ctrl Pts',(-2.49999999999999,1.33275179473161,-66.));
#33690=CARTESIAN_POINT('Ctrl Pts',(-2.42122743991223,0.985650418224739,
-65.9509027104217));
#33691=CARTESIAN_POINT('Ctrl Pts',(-1.89279714334289,0.308835349231178,
-65.5507400778319));
#33692=CARTESIAN_POINT('Ctrl Pts',(-1.24643975969902,0.0209726669473527,
-64.9588414442702));
#33693=CARTESIAN_POINT('Ctrl Pts',(-0.868245358015784,0.00185294611160958,
-64.5745345887862));
#33694=CARTESIAN_POINT('Origin',(-2.75,4.,-65.75));
#33695=CARTESIAN_POINT('',(-3.,4.,-65.5));
#33696=CARTESIAN_POINT('',(-2.5,4.,-66.));
#33697=CARTESIAN_POINT('',(-14.375,4.,-54.125));
#33698=CARTESIAN_POINT('',(-2.5,4.,-66.));
#33699=CARTESIAN_POINT('',(-3.,4.,-65.5));
#33700=CARTESIAN_POINT('Origin',(0.,0.,-16.5));
#33701=CARTESIAN_POINT('',(-38.,0.,42.));
#33702=CARTESIAN_POINT('',(-17.5,0.,42.));
#33703=CARTESIAN_POINT('',(-19.,0.,42.));
#33704=CARTESIAN_POINT('',(-64.5,0.,15.5));
#33705=CARTESIAN_POINT('Origin',(-38.,0.,15.5));
#33706=CARTESIAN_POINT('',(-64.5,0.,-48.5));
#33707=CARTESIAN_POINT('',(-64.5,0.,-32.5));
#33708=CARTESIAN_POINT('',(-38.,0.,-75.));
#33709=CARTESIAN_POINT('Origin',(-38.,0.,-48.5));
#33710=CARTESIAN_POINT('',(38.,0.,-75.));
#33711=CARTESIAN_POINT('',(19.,0.,-75.));
#33712=CARTESIAN_POINT('',(64.5,0.,-48.5));
#33713=CARTESIAN_POINT('Origin',(38.,0.,-48.5));
#33714=CARTESIAN_POINT('',(64.5,0.,15.5));
#33715=CARTESIAN_POINT('',(64.5,0.,-0.500000000000003));
#33716=CARTESIAN_POINT('',(38.,0.,42.));
#33717=CARTESIAN_POINT('Origin',(38.,0.,15.5));
#33718=CARTESIAN_POINT('',(17.5,0.,42.));
#33719=CARTESIAN_POINT('',(-19.,0.,42.));
#33720=CARTESIAN_POINT('Origin',(0.,0.,0.));
#33721=CARTESIAN_POINT('',(47.2,0.,-7.34788079488411E-16));
#33722=CARTESIAN_POINT('Origin',(53.2,0.,0.));
#33723=CARTESIAN_POINT('',(0.795318636409267,0.,-64.5));
#33724=CARTESIAN_POINT('',(-1.5,0.,-64.5));
#33725=CARTESIAN_POINT('',(1.5,0.,-63.7953186364093));
#33726=CARTESIAN_POINT('',(1.14765931820464,0.,-64.1476593182046));
#33727=CARTESIAN_POINT('',(1.50000000000001,0.,-45.4752680036083));
#33728=CARTESIAN_POINT('',(1.5,0.,-41.25));
#33729=CARTESIAN_POINT('',(31.0952102098472,0.,-33.2165305534069));
#33730=CARTESIAN_POINT('Origin',(0.,0.,0.));
#33731=CARTESIAN_POINT('',(45.2548339959391,0.,-47.3761543394987));
#33732=CARTESIAN_POINT('',(18.6206890143242,0.,-20.7420093578839));
#33733=CARTESIAN_POINT('',(47.3761543394987,0.,-45.254833995939));
#33734=CARTESIAN_POINT('',(41.129833995939,0.,-51.5011543394987));
#33735=CARTESIAN_POINT('',(33.2165305534069,0.,-31.0952102098472));
#33736=CARTESIAN_POINT('',(28.5201839509359,0.,-26.3988636073762));
#33737=CARTESIAN_POINT('',(45.209022556391,0.,-5.13753632549022));
#33738=CARTESIAN_POINT('Origin',(0.,0.,0.));
#33739=CARTESIAN_POINT('',(59.5,0.,-7.11055553385247));
#33740=CARTESIAN_POINT('Origin',(53.2,0.,0.));
#33741=CARTESIAN_POINT('',(59.5,0.,-46.5));
#33742=CARTESIAN_POINT('',(59.5,0.,-1.5));
#33743=CARTESIAN_POINT('',(36.,0.,-70.));
#33744=CARTESIAN_POINT('Origin',(36.,0.,-46.5));
#33745=CARTESIAN_POINT('',(-36.,0.,-70.));
#33746=CARTESIAN_POINT('',(18.,0.,-70.));
#33747=CARTESIAN_POINT('',(-59.5,0.,-46.5));
#33748=CARTESIAN_POINT('Origin',(-36.,0.,-46.5));
#33749=CARTESIAN_POINT('',(-59.5,0.,-7.11055553385247));
#33750=CARTESIAN_POINT('',(-59.5,0.,-31.5));
#33751=CARTESIAN_POINT('',(-45.209022556391,0.,-5.13753632549022));
#33752=CARTESIAN_POINT('Origin',(-53.2,0.,0.));
#33753=CARTESIAN_POINT('',(-33.2165305534069,0.,-31.0952102098472));
#33754=CARTESIAN_POINT('Origin',(0.,0.,0.));
#33755=CARTESIAN_POINT('',(-46.1707625875413,0.,-44.0494422439817));
#33756=CARTESIAN_POINT('',(-20.7420093578839,0.,-18.6206890143242));
#33757=CARTESIAN_POINT('',(-46.1707625875413,0.,-45.0460121855233));
#33758=CARTESIAN_POINT('',(-46.1707625875413,0.,-44.5477272147525));
#33759=CARTESIAN_POINT('',(-45.0460121855233,0.,-46.1707625875413));
#33760=CARTESIAN_POINT('',(-42.5440475583121,0.,-48.6727272147525));
#33761=CARTESIAN_POINT('',(-44.0494422439817,0.,-46.1707625875413));
#33762=CARTESIAN_POINT('',(-44.5477272147525,0.,-46.1707625875413));
#33763=CARTESIAN_POINT('',(-31.0952102098472,0.,-33.2165305534069));
#33764=CARTESIAN_POINT('',(-26.3988636073762,0.,-28.5201839509359));
#33765=CARTESIAN_POINT('',(-1.49999999999998,0.,-45.4752680036083));
#33766=CARTESIAN_POINT('Origin',(0.,0.,0.));
#33767=CARTESIAN_POINT('',(-1.5,0.,-30.25));
#33768=CARTESIAN_POINT('',(59.5,0.,13.5));
#33769=CARTESIAN_POINT('',(36.,0.,37.));
#33770=CARTESIAN_POINT('Origin',(36.,0.,13.5));
#33771=CARTESIAN_POINT('',(59.5,0.,7.11055553385247));
#33772=CARTESIAN_POINT('',(59.5,0.,-1.5));
#33773=CARTESIAN_POINT('',(45.209022556391,0.,5.13753632549028));
#33774=CARTESIAN_POINT('Origin',(53.2,0.,0.));
#33775=CARTESIAN_POINT('',(26.4811253537307,0.,37.));
#33776=CARTESIAN_POINT('Origin',(0.,0.,0.));
#33777=CARTESIAN_POINT('',(-18.,0.,37.));
#33778=CARTESIAN_POINT('',(36.4780836837786,0.,19.3232453474888));
#33779=CARTESIAN_POINT('',(29.8463073008423,0.,28.5172989692869));
#33780=CARTESIAN_POINT('Origin',(30.5,0.,22.));
#33781=CARTESIAN_POINT('',(-5.05534198688027E-15,0.,-41.28));
#33782=CARTESIAN_POINT('Origin',(0.,0.,0.));
#33783=CARTESIAN_POINT('',(-36.4780836837786,0.,19.3232453474888));
#33784=CARTESIAN_POINT('Origin',(0.,0.,0.));
#33785=CARTESIAN_POINT('',(-29.8463073008423,0.,28.5172989692869));
#33786=CARTESIAN_POINT('Origin',(-30.5,0.,22.));
#33787=CARTESIAN_POINT('Origin',(0.,0.,0.));
#33788=CARTESIAN_POINT('',(-36.,0.,37.));
#33789=CARTESIAN_POINT('',(-59.5,0.,13.5));
#33790=CARTESIAN_POINT('Origin',(-36.,0.,13.5));
#33791=CARTESIAN_POINT('',(-26.4811253537307,0.,37.));
#33792=CARTESIAN_POINT('',(-18.,0.,37.));
#33793=CARTESIAN_POINT('',(-45.209022556391,0.,5.13753632549025));
#33794=CARTESIAN_POINT('Origin',(0.,0.,0.));
#33795=CARTESIAN_POINT('',(-59.5,0.,7.11055553385247));
#33796=CARTESIAN_POINT('Origin',(-53.2,0.,0.));
#33797=CARTESIAN_POINT('',(-59.5,0.,-31.5));
#33798=CARTESIAN_POINT('',(-59.2,0.,-7.34788079488411E-16));
#33799=CARTESIAN_POINT('Origin',(-53.2,0.,0.));
#33800=CARTESIAN_POINT('Origin',(-1.5,1.5,-64.5));
#33801=CARTESIAN_POINT('',(2.5,1.5,-66.));
#33802=CARTESIAN_POINT('',(-1.5,1.5,-66.));
#33803=CARTESIAN_POINT('',(0.868245358015795,0.00185294611160958,-64.5745345887862));
#33804=CARTESIAN_POINT('Ctrl Pts',(0.868245358015795,0.00185294611160958,
-64.5745345887862));
#33805=CARTESIAN_POINT('Ctrl Pts',(1.12037495913795,0.0145994266687717,
-64.8307391591089));
#33806=CARTESIAN_POINT('Ctrl Pts',(1.63375136411347,0.173220581778977,-65.3201513636217));
#33807=CARTESIAN_POINT('Ctrl Pts',(2.13540546748456,0.600909021307247,-65.7357961587963));
#33808=CARTESIAN_POINT('Ctrl Pts',(2.43900967406247,1.07263972227481,-65.9615334712268));
#33809=CARTESIAN_POINT('Ctrl Pts',(2.5,1.33275179473161,-66.));
#33810=CARTESIAN_POINT('Ctrl Pts',(2.5,1.5,-66.));
#33811=CARTESIAN_POINT('Ctrl Pts',(0.795318636409267,-2.22044604925031E-16,
-64.5));
#33812=CARTESIAN_POINT('Ctrl Pts',(0.795642656641266,-2.22020079281761E-16,
-64.5003313610337));
#33813=CARTESIAN_POINT('Ctrl Pts',(0.795969871010492,9.12216844667872E-8,
-64.5006659910395));
#33814=CARTESIAN_POINT('Ctrl Pts',(0.796372819533867,3.87472611551587E-7,
-64.5010781547591));
#33815=CARTESIAN_POINT('Ctrl Pts',(0.79679572105221,6.98393137642135E-7,
-64.501510727787));
#33816=CARTESIAN_POINT('Ctrl Pts',(0.797301839401443,1.2319450398306E-6,
-64.5020284953742));
#33817=CARTESIAN_POINT('Ctrl Pts',(0.797934442187392,2.38657547613208E-6,
-64.502675765448));
#33818=CARTESIAN_POINT('Ctrl Pts',(0.798608415722088,3.61671605360927E-6,
-64.5033653654769));
#33819=CARTESIAN_POINT('Ctrl Pts',(0.799425679468639,5.55516755123648E-6,
-64.5042016754148));
#33820=CARTESIAN_POINT('Ctrl Pts',(0.800397213439585,8.99934440856676E-6,
-64.505195955373));
#33821=CARTESIAN_POINT('Ctrl Pts',(0.801469705844418,1.28014281553561E-5,
-64.5062935574489));
#33822=CARTESIAN_POINT('Ctrl Pts',(0.802729790879233,1.84658046873067E-5,
-64.5075832522893));
#33823=CARTESIAN_POINT('Ctrl Pts',(0.804148443709076,2.72127176239589E-5,
-64.5090353424031));
#33824=CARTESIAN_POINT('Ctrl Pts',(0.805928294908851,3.81866523013816E-5,
-64.5108571442398));
#33825=CARTESIAN_POINT('Ctrl Pts',(0.807956854596668,5.41281456196828E-5,
-64.5129336615424));
#33826=CARTESIAN_POINT('Ctrl Pts',(0.810118702324731,7.64762491842763E-5,
-64.5151467124795));
#33827=CARTESIAN_POINT('Ctrl Pts',(0.812412161386584,0.000100184885074821,
-64.5174944919555));
#33828=CARTESIAN_POINT('Ctrl Pts',(0.814850893768659,0.000131146817813719,
-64.5199910876103));
#33829=CARTESIAN_POINT('Ctrl Pts',(0.817286906240445,0.000168532538717292,
-64.522484866309));
#33830=CARTESIAN_POINT('Ctrl Pts',(0.819132499158045,0.000196857033159806,
-64.524374224577));
#33831=CARTESIAN_POINT('Ctrl Pts',(0.82097572933093,0.000228767928633297,
-64.5262611440487));
#33832=CARTESIAN_POINT('Ctrl Pts',(0.82277575793104,0.000263295917060091,
-64.5281037084108));
#33833=CARTESIAN_POINT('Ctrl Pts',(0.824400036902089,0.000294452691741817,
-64.5297663700741));
#33834=CARTESIAN_POINT('Ctrl Pts',(0.82598873685544,0.000327690884686428,
-64.531392504458));
#33835=CARTESIAN_POINT('Ctrl Pts',(0.827540750553837,0.000362622665139645,
-64.5329808505079));
#33836=CARTESIAN_POINT('Ctrl Pts',(0.82907180232416,0.000397082647263948,
-64.5345477439148));
#33837=CARTESIAN_POINT('Ctrl Pts',(0.830566495721296,0.000433137034785286,
-64.5360771924232));
#33838=CARTESIAN_POINT('Ctrl Pts',(0.832061473905696,0.000471490904882854,
-64.5376065208571));
#33839=CARTESIAN_POINT('Ctrl Pts',(0.833519495899744,0.000508896658854833,
-64.5390980439549));
#33840=CARTESIAN_POINT('Ctrl Pts',(0.834984333446768,0.000548663598861856,
-64.5405961355826));
#33841=CARTESIAN_POINT('Ctrl Pts',(0.836485232609497,0.000591779397116854,
-64.5421306063153));
#33842=CARTESIAN_POINT('Ctrl Pts',(0.838098400887085,0.000638120310440689,
-64.5437798573578));
#33843=CARTESIAN_POINT('Ctrl Pts',(0.839752877016141,0.000688360290152621,
-64.5454707747875));
#33844=CARTESIAN_POINT('Ctrl Pts',(0.841442884797579,0.00074271667356185,
-64.5471974405305));
#33845=CARTESIAN_POINT('Ctrl Pts',(0.843373591615611,0.000804814754531903,
-64.5491700263133));
#33846=CARTESIAN_POINT('Ctrl Pts',(0.845350148493538,0.000872336312437336,
-64.5511887316101));
#33847=CARTESIAN_POINT('Ctrl Pts',(0.847317128680503,0.000943604228316186,
-64.5531970139764));
#33848=CARTESIAN_POINT('Ctrl Pts',(0.850042283731077,0.00104234244753579,
-64.5559793911808));
#33849=CARTESIAN_POINT('Ctrl Pts',(0.852746171331635,0.00114840209592096,
-64.5587388045197));
#33850=CARTESIAN_POINT('Ctrl Pts',(0.855216138687543,0.00125139174845401,
-64.5612585444167));
#33851=CARTESIAN_POINT('Ctrl Pts',(0.857068614204475,0.0013286339878538,
-64.5631483493395));
#33852=CARTESIAN_POINT('Ctrl Pts',(0.858786862306446,0.00140389724195783,
-64.5649006457068));
#33853=CARTESIAN_POINT('Ctrl Pts',(0.860296358541392,0.00147212889990866,
-64.5664395931371));
#33854=CARTESIAN_POINT('Ctrl Pts',(0.861561043718845,0.00152929470426492,
-64.5677289530964));
#33855=CARTESIAN_POINT('Ctrl Pts',(0.862678831397432,0.00158146111031607,
-64.5688681843539));
#33856=CARTESIAN_POINT('Ctrl Pts',(0.863631665321587,0.00162671007902326,
-64.5698389866149));
#33857=CARTESIAN_POINT('Ctrl Pts',(0.864527500020132,0.00166925222116752,
-64.5707517147711));
#33858=CARTESIAN_POINT('Ctrl Pts',(0.865277115559362,0.00170564250683912,
-64.5715151450229));
#33859=CARTESIAN_POINT('Ctrl Pts',(0.865895865152574,0.00173597254573621,
-64.5721450208714));
#33860=CARTESIAN_POINT('Ctrl Pts',(0.866472565487434,0.00176424140244366,
-64.5727320913385));
#33861=CARTESIAN_POINT('Ctrl Pts',(0.866935434874884,0.00178723762245152,
-64.5732029927807));
#33862=CARTESIAN_POINT('Ctrl Pts',(0.867327729258992,0.00180683428705319,
-64.5736018899962));
#33863=CARTESIAN_POINT('Ctrl Pts',(0.867669871372873,0.00182392564630644,
-64.5739497908127));
#33864=CARTESIAN_POINT('Ctrl Pts',(0.867958593712563,0.00183844866426747,
-64.5742431897408));
#33865=CARTESIAN_POINT('Ctrl Pts',(0.868245358015795,0.00185294611160947,
-64.5745345887863));
#33866=CARTESIAN_POINT('Origin',(-3.,4.,-66.));
#33867=CARTESIAN_POINT('',(2.5,4.,-66.));
#33868=CARTESIAN_POINT('',(-1.5,4.,-66.));
#33869=CARTESIAN_POINT('',(2.5,4.,-66.));
#33870=CARTESIAN_POINT('Ctrl Pts',(0.868245358015795,0.00185294611160958,
-64.5745345887862));
#33871=CARTESIAN_POINT('Ctrl Pts',(0.864163358505955,0.00164657951619623,
-64.5703866151813));
#33872=CARTESIAN_POINT('Ctrl Pts',(0.834260393339435,0.000219540540015439,
-64.539887259118));
#33873=CARTESIAN_POINT('Ctrl Pts',(0.801608171182561,1.28888202263847E-5,
-64.5064246347597));
#33874=CARTESIAN_POINT('Ctrl Pts',(0.796336597880222,9.63140470631229E-20,
-64.5010410237755));
#33875=CARTESIAN_POINT('Ctrl Pts',(0.795318636409267,0.,-64.5));
#33876=CARTESIAN_POINT('Ctrl Pts',(1.10367510160595,0.00185294611160967,
-64.3391048451961));
#33877=CARTESIAN_POINT('Ctrl Pts',(1.09957111073108,0.0016465795161963,
-64.3349788629562));
#33878=CARTESIAN_POINT('Ctrl Pts',(1.06943670599212,0.000219540540015618,
-64.3047109464653));
#33879=CARTESIAN_POINT('Ctrl Pts',(1.03655657695391,1.28888202263034E-5,
-64.2714762289883));
#33880=CARTESIAN_POINT('Ctrl Pts',(1.03123807317865,2.26183380401734E-19,
-64.2661395484771));
#33881=CARTESIAN_POINT('Ctrl Pts',(1.03021242427285,0.,-64.2651062121364));
#33882=CARTESIAN_POINT('Ctrl Pts',(1.33910484519611,0.00185294611160976,
-64.1036751016059));
#33883=CARTESIAN_POINT('Ctrl Pts',(1.33497886295621,0.0016465795161964,
-64.0995711107311));
#33884=CARTESIAN_POINT('Ctrl Pts',(1.30453395202334,-2.1594682714537E-5,
-64.0694367059921));
#33885=CARTESIAN_POINT('Ctrl Pts',(1.27145164420996,0.000165305522379591,
-64.0365565769539));
#33886=CARTESIAN_POINT('Ctrl Pts',(1.26613954847709,3.59888273472094E-19,
-64.0312380731786));
#33887=CARTESIAN_POINT('Ctrl Pts',(1.26510621213642,0.,-64.0302124242728));
#33888=CARTESIAN_POINT('Ctrl Pts',(1.57453458878627,0.00185294611160985,
-63.8682453580158));
#33889=CARTESIAN_POINT('Ctrl Pts',(1.57038661518134,0.0016465795161965,
-63.8641633585059));
#33890=CARTESIAN_POINT('Ctrl Pts',(1.539887259118,0.000219540540015942,
-63.8342603933394));
#33891=CARTESIAN_POINT('Ctrl Pts',(1.5064246347597,1.28888202263958E-5,
-63.8016081711826));
#33892=CARTESIAN_POINT('Ctrl Pts',(1.50104102377552,4.81570235315835E-19,
-63.7963365978802));
#33893=CARTESIAN_POINT('Ctrl Pts',(1.5,0.,-63.7953186364093));
#33894=CARTESIAN_POINT('',(1.57453458878627,0.00185294611160985,-63.8682453580158));
#33895=CARTESIAN_POINT('Ctrl Pts',(1.57453458878627,0.00185294611160985,
-63.8682453580158));
#33896=CARTESIAN_POINT('Ctrl Pts',(1.33910484519611,0.00185294611160976,
-64.1036751016059));
#33897=CARTESIAN_POINT('Ctrl Pts',(1.10367510160595,0.00185294611160967,
-64.3391048451961));
#33898=CARTESIAN_POINT('Ctrl Pts',(0.868245358015795,0.00185294611160958,
-64.5745345887862));
#33899=CARTESIAN_POINT('Ctrl Pts',(1.57453458878627,0.00185294611160969,
-63.8682453580158));
#33900=CARTESIAN_POINT('Ctrl Pts',(1.57420449252805,0.00183652343213895,
-63.8679205119843));
#33901=CARTESIAN_POINT('Ctrl Pts',(1.57387113100176,0.00182002913551295,
-63.8675924675611));
#33902=CARTESIAN_POINT('Ctrl Pts',(1.57346041281005,0.00179989061882035,
-63.867188603525));
#33903=CARTESIAN_POINT('Ctrl Pts',(1.57302935509002,0.0017787548053465,
-63.8667647393911));
#33904=CARTESIAN_POINT('Ctrl Pts',(1.57251329683896,0.00175361200744156,
-63.8662575638241));
#33905=CARTESIAN_POINT('Ctrl Pts',(1.57186801151716,0.00172265954511253,
-63.8656237691205));
#33906=CARTESIAN_POINT('Ctrl Pts',(1.57118052112909,0.00168968262836032,
-63.8649485208977));
#33907=CARTESIAN_POINT('Ctrl Pts',(1.5703466306137,0.0016501286772923,-63.8641298278249));
#33908=CARTESIAN_POINT('Ctrl Pts',(1.56935505358675,0.00160423233980667,
-63.8631567176194));
#33909=CARTESIAN_POINT('Ctrl Pts',(1.56826041042658,0.00155356546215597,
-63.8620824607523));
#33910=CARTESIAN_POINT('Ctrl Pts',(1.56697400911583,0.00149521701852808,
-63.8608204240659));
#33911=CARTESIAN_POINT('Ctrl Pts',(1.56552538795896,0.00143187557828095,
-63.8593997067428));
#33912=CARTESIAN_POINT('Ctrl Pts',(1.56370772709104,0.00135239775434526,
-63.8576170582771));
#33913=CARTESIAN_POINT('Ctrl Pts',(1.56163556088225,0.0012652187682126,
-63.8555854664071));
#33914=CARTESIAN_POINT('Ctrl Pts',(1.55942667679053,0.00117763891592682,
-63.8534206289471));
#33915=CARTESIAN_POINT('Ctrl Pts',(1.55708422198041,0.00108476312990192,
-63.8511248842586));
#33916=CARTESIAN_POINT('Ctrl Pts',(1.55459284718984,0.000991719524377037,
-63.8486840335238));
#33917=CARTESIAN_POINT('Ctrl Pts',(1.55210358759418,0.000905201076390805,
-63.8462462517521));
#33918=CARTESIAN_POINT('Ctrl Pts',(1.55021730688321,0.000839640184363255,
-63.8443989792773));
#33919=CARTESIAN_POINT('Ctrl Pts',(1.54833306473991,0.000777766532137521,
-63.8425542719585));
#33920=CARTESIAN_POINT('Ctrl Pts',(1.54649262612169,0.000720694561447077,
-63.8407530639427));
#33921=CARTESIAN_POINT('Ctrl Pts',(1.54483185722751,0.000669194145886256,
-63.8391276958293));
#33922=CARTESIAN_POINT('Ctrl Pts',(1.54320716885208,0.000621574660657379,
-63.8375381508115));
#33923=CARTESIAN_POINT('Ctrl Pts',(1.54161975843489,0.000577512604328589,
-63.8359855786446));
#33924=CARTESIAN_POINT('Ctrl Pts',(1.54005331925714,0.000534032650727231,
-63.8344535174698));
#33925=CARTESIAN_POINT('Ctrl Pts',(1.53852385337071,0.000493996445439231,
-63.8329581182172));
#33926=CARTESIAN_POINT('Ctrl Pts',(1.53699396768853,0.000456253937664908,
-63.8314627005844));
#33927=CARTESIAN_POINT('Ctrl Pts',(1.53550237601382,0.000419456148761565,
-63.830004714202));
#33928=CARTESIAN_POINT('Ctrl Pts',(1.53400370375587,0.000384680303817308,
-63.8285401666312));
#33929=CARTESIAN_POINT('Ctrl Pts',(1.53246818059487,0.000351435419331247,
-63.8270398157865));
#33930=CARTESIAN_POINT('Ctrl Pts',(1.53081777199523,0.000315703204641898,
-63.8254272110409));
#33931=CARTESIAN_POINT('Ctrl Pts',(1.52912514926818,0.000281787957712134,
-63.8237735951328));
#33932=CARTESIAN_POINT('Ctrl Pts',(1.52739631907099,0.000250206967388422,
-63.8220847050031));
#33933=CARTESIAN_POINT('Ctrl Pts',(1.52542113854251,0.000214125831566566,
-63.8201551558176));
#33934=CARTESIAN_POINT('Ctrl Pts',(1.52339923128973,0.00018116946976938,
-63.818180086159));
#33935=CARTESIAN_POINT('Ctrl Pts',(1.52138736276008,0.00015248084541275,
-63.8162148275183));
#33936=CARTESIAN_POINT('Ctrl Pts',(1.51860054020794,0.000112741615851503,
-63.8134925685733));
#33937=CARTESIAN_POINT('Ctrl Pts',(1.51583593600687,8.14691463204668E-5,
-63.8107920180653));
#33938=CARTESIAN_POINT('Ctrl Pts',(1.51331094781377,5.90616066578065E-5,
-63.8083253911404));
#33939=CARTESIAN_POINT('Ctrl Pts',(1.51141720666895,4.22559519108112E-5,
-63.8064754209468));
#33940=CARTESIAN_POINT('Ctrl Pts',(1.50966095085537,3.03183594527219E-5,
-63.8047596756712));
#33941=CARTESIAN_POINT('Ctrl Pts',(1.50811830943101,2.19691435532354E-5,
-63.803252515256));
#33942=CARTESIAN_POINT('Ctrl Pts',(1.50682582394888,1.49738430467655E-5,
-63.8019897571548));
#33943=CARTESIAN_POINT('Ctrl Pts',(1.5056836631397,1.04521897692208E-5,
-63.8008737857751));
#33944=CARTESIAN_POINT('Ctrl Pts',(1.50471023759975,7.39546431272053E-6,
-63.7999226003202));
#33945=CARTESIAN_POINT('Ctrl Pts',(1.50379503110595,4.521556784394E-6,-63.7990283037671));
#33946=CARTESIAN_POINT('Ctrl Pts',(1.50302939881844,2.92603171356413E-6,
-63.79828008132));
#33947=CARTESIAN_POINT('Ctrl Pts',(1.50239760011449,1.91616332689826E-6,
-63.797662574869));
#33948=CARTESIAN_POINT('Ctrl Pts',(1.50180873020872,9.74912422190382E-7,
-63.7970870261012));
#33949=CARTESIAN_POINT('Ctrl Pts',(1.50133627503617,5.41797940298606E-7,
-63.7966251806828));
#33950=CARTESIAN_POINT('Ctrl Pts',(1.50093597841904,2.92018561776075E-7,
-63.7962338194152));
#33951=CARTESIAN_POINT('Ctrl Pts',(1.50058692053362,7.42114208744582E-8,
-63.7958925531375));
#33952=CARTESIAN_POINT('Ctrl Pts',(1.50029246039094,-2.2193637283843E-16,
-63.7956046177833));
#33953=CARTESIAN_POINT('Ctrl Pts',(1.5,-2.22044604925031E-16,-63.7953186364093));
#33954=CARTESIAN_POINT('Ctrl Pts',(1.57453458878627,0.00185294611160985,
-63.8682453580158));
#33955=CARTESIAN_POINT('Ctrl Pts',(1.83073915910892,0.0145994266687731,
-64.1203749591379));
#33956=CARTESIAN_POINT('Ctrl Pts',(2.32015136362177,0.173220581778977,-64.6337513641135));
#33957=CARTESIAN_POINT('Ctrl Pts',(2.73579615879626,0.600909021307247,-65.1354054674845));
#33958=CARTESIAN_POINT('Ctrl Pts',(2.96153347122678,1.07263972227482,-65.4390096740624));
#33959=CARTESIAN_POINT('Ctrl Pts',(3.,1.33275179473161,-65.5));
#33960=CARTESIAN_POINT('Ctrl Pts',(3.,1.5,-65.5));
#33961=CARTESIAN_POINT('Ctrl Pts',(1.33910484519611,0.00185294611160976,
-64.1036751016059));
#33962=CARTESIAN_POINT('Ctrl Pts',(1.59395109245193,0.0145994266687726,
-64.3571630257949));
#33963=CARTESIAN_POINT('Ctrl Pts',(2.09135136378567,0.173220581778977,-64.8625513639496));
#33964=CARTESIAN_POINT('Ctrl Pts',(2.53566592835903,0.600909021307248,-65.3355356979218));
#33965=CARTESIAN_POINT('Ctrl Pts',(2.78735887217201,1.07263972227482,-65.6131842731172));
#33966=CARTESIAN_POINT('Ctrl Pts',(2.83333333333334,1.33275179473161,-65.6666666666667));
#33967=CARTESIAN_POINT('Ctrl Pts',(2.83333333333334,1.5,-65.6666666666667));
#33968=CARTESIAN_POINT('Ctrl Pts',(1.10367510160595,0.00185294611160967,
-64.3391048451961));
#33969=CARTESIAN_POINT('Ctrl Pts',(1.35716302579494,0.0145994266687722,
-64.5939510924519));
#33970=CARTESIAN_POINT('Ctrl Pts',(1.86255136394957,0.173220581778978,-65.0913513637857));
#33971=CARTESIAN_POINT('Ctrl Pts',(2.33553569792179,0.600909021307247,-65.535665928359));
#33972=CARTESIAN_POINT('Ctrl Pts',(2.61318427311724,1.07263972227482,-65.787358872172));
#33973=CARTESIAN_POINT('Ctrl Pts',(2.66666666666667,1.33275179473161,-65.8333333333333));
#33974=CARTESIAN_POINT('Ctrl Pts',(2.66666666666667,1.5,-65.8333333333333));
#33975=CARTESIAN_POINT('Ctrl Pts',(0.868245358015795,0.00185294611160958,
-64.5745345887862));
#33976=CARTESIAN_POINT('Ctrl Pts',(1.12037495913795,0.0145994266687717,
-64.8307391591089));
#33977=CARTESIAN_POINT('Ctrl Pts',(1.63375136411347,0.173220581778977,-65.3201513636217));
#33978=CARTESIAN_POINT('Ctrl Pts',(2.13540546748456,0.600909021307247,-65.7357961587963));
#33979=CARTESIAN_POINT('Ctrl Pts',(2.43900967406247,1.07263972227481,-65.9615334712268));
#33980=CARTESIAN_POINT('Ctrl Pts',(2.5,1.33275179473161,-66.));
#33981=CARTESIAN_POINT('Ctrl Pts',(2.5,1.5,-66.));
#33982=CARTESIAN_POINT('',(3.,1.5,-65.5));
#33983=CARTESIAN_POINT('',(2.5,1.5,-66.));
#33984=CARTESIAN_POINT('Ctrl Pts',(3.,1.5,-65.5));
#33985=CARTESIAN_POINT('Ctrl Pts',(3.,1.33275179473161,-65.5));
#33986=CARTESIAN_POINT('Ctrl Pts',(2.96153347122678,1.07263972227482,-65.4390096740624));
#33987=CARTESIAN_POINT('Ctrl Pts',(2.73579615879626,0.600909021307247,-65.1354054674845));
#33988=CARTESIAN_POINT('Ctrl Pts',(2.32015136362177,0.173220581778977,-64.6337513641135));
#33989=CARTESIAN_POINT('Ctrl Pts',(1.83073915910892,0.0145994266687731,
-64.1203749591379));
#33990=CARTESIAN_POINT('Ctrl Pts',(1.57453458878627,0.00185294611160985,
-63.8682453580158));
#33991=CARTESIAN_POINT('Origin',(2.75,4.,-65.75));
#33992=CARTESIAN_POINT('',(3.,4.,-65.5));
#33993=CARTESIAN_POINT('',(14.375,4.,-54.1249999999998));
#33994=CARTESIAN_POINT('',(3.,4.,-65.5));
#33995=CARTESIAN_POINT('Origin',(1.5,1.5,-41.25));
#33996=CARTESIAN_POINT('',(3.,1.5,-46.9041575982343));
#33997=CARTESIAN_POINT('',(3.,1.5,-41.25));
#33998=CARTESIAN_POINT('Ctrl Pts',(3.,1.5,-46.9041575982343));
#33999=CARTESIAN_POINT('Ctrl Pts',(3.,1.35551296703019,-46.9041575982343));
#34000=CARTESIAN_POINT('Ctrl Pts',(2.97913882256008,1.2141617946757,-46.8845984232444));
#34001=CARTESIAN_POINT('Ctrl Pts',(2.89577102625226,0.928389940435113,-46.8062984441602));
#34002=CARTESIAN_POINT('Ctrl Pts',(2.82982150540341,0.791053413169228,-46.7443046032146));
#34003=CARTESIAN_POINT('Ctrl Pts',(2.64514766490965,0.512937531198892,-46.5701910337406));
#34004=CARTESIAN_POINT('Ctrl Pts',(2.51762496582942,0.38503558873678,-46.4496283712152));
#34005=CARTESIAN_POINT('Ctrl Pts',(2.24921701551044,0.190439066398323,-46.1946602843644));
#34006=CARTESIAN_POINT('Ctrl Pts',(2.10792859962105,0.120380195566533,-46.059925664155));
#34007=CARTESIAN_POINT('Ctrl Pts',(1.81376170731678,0.024706643928065,-45.7780704433202));
#34008=CARTESIAN_POINT('Ctrl Pts',(1.65894854459693,0.000552890155855622,
-45.6290430115594));
#34009=CARTESIAN_POINT('Ctrl Pts',(1.50353740181663,3.12821524572435E-6,
-45.4786905515984));
#34010=CARTESIAN_POINT('Ctrl Pts',(1.50176867612926,1.08300178020774E-19,
-45.4769793019272));
#34011=CARTESIAN_POINT('Ctrl Pts',(1.50000000000001,0.,-45.4752680036083));
#34012=CARTESIAN_POINT('Origin',(3.,4.,-66.));
#34013=CARTESIAN_POINT('',(3.,4.,-46.9041575982343));
#34014=CARTESIAN_POINT('',(3.,4.,-41.25));
#34015=CARTESIAN_POINT('',(3.,4.,-46.9041575982343));
#34016=CARTESIAN_POINT('Origin',(-30.5,0.25,-55.));
#34017=CARTESIAN_POINT('',(-35.55,0.5,-55.));
#34018=CARTESIAN_POINT('',(-35.8,0.25,-55.));
#34019=CARTESIAN_POINT('Origin',(-30.5,0.5,-55.));
#34020=CARTESIAN_POINT('Origin',(-30.5,18.,-55.));
#34021=CARTESIAN_POINT('',(-35.55,17.5,-55.));
#34022=CARTESIAN_POINT('Origin',(-30.5,17.5,-55.));
#34023=CARTESIAN_POINT('',(-35.55,18.,-55.));
#34024=CARTESIAN_POINT('Origin',(30.5,0.25,-55.));
#34025=CARTESIAN_POINT('',(25.45,0.5,-55.));
#34026=CARTESIAN_POINT('',(25.2,0.25,-55.));
#34027=CARTESIAN_POINT('Origin',(30.5,0.5,-55.));
#34028=CARTESIAN_POINT('Origin',(30.5,18.,-55.));
#34029=CARTESIAN_POINT('',(25.45,17.5,-55.));
#34030=CARTESIAN_POINT('Origin',(30.5,17.5,-55.));
#34031=CARTESIAN_POINT('',(25.45,18.,-55.));
#34032=CARTESIAN_POINT('Origin',(35.5422371315094,-2.7,20.6547211791723));
#34033=CARTESIAN_POINT('',(35.7247978384185,0.551098954346127,20.682775911471));
#34034=CARTESIAN_POINT('',(35.3596764246032,1.5,20.6266664468687));
#34035=CARTESIAN_POINT('Ctrl Pts',(35.3596764246032,1.5,20.6266664468687));
#34036=CARTESIAN_POINT('Ctrl Pts',(35.3596764246032,1.31962574714054,20.6266664468687));
#34037=CARTESIAN_POINT('Ctrl Pts',(35.40452588567,1.10798634108372,20.6335586179471));
#34038=CARTESIAN_POINT('Ctrl Pts',(35.5338848608011,0.809115390967544,20.6534376569795));
#34039=CARTESIAN_POINT('Ctrl Pts',(35.6230425085747,0.667215858409758,20.667138819642));
#34040=CARTESIAN_POINT('Ctrl Pts',(35.7247978384207,0.551098954350102,20.6827759114767));
#34041=CARTESIAN_POINT('',(35.3596764208672,-0.844289827423071,20.6266664336486));
#34042=CARTESIAN_POINT('',(35.3596764246032,-2.7,20.6266664468687));
#34043=CARTESIAN_POINT('',(35.7247978384157,-1.8,20.6827759114759));
#34044=CARTESIAN_POINT('Ctrl Pts',(35.7247978384157,-1.8,20.6827759114759));
#34045=CARTESIAN_POINT('Ctrl Pts',(35.7247978384157,-1.61916866909503,20.6827759114759));
#34046=CARTESIAN_POINT('Ctrl Pts',(35.6808305167185,-1.40677945093785,20.6760193017913));
#34047=CARTESIAN_POINT('Ctrl Pts',(35.552259697619,-1.10534194031554,20.6562613814095));
#34048=CARTESIAN_POINT('Ctrl Pts',(35.4623482875555,-0.961189978401695,
20.642444385501));
#34049=CARTESIAN_POINT('Ctrl Pts',(35.3596764103059,-0.84428983506834,20.6266664446716));
#34050=CARTESIAN_POINT('',(35.7247978384157,-2.7,20.6827759114759));
#34051=CARTESIAN_POINT('Origin',(30.5,18.,22.));
#34052=CARTESIAN_POINT('',(25.45,17.5,22.));
#34053=CARTESIAN_POINT('Origin',(30.5,17.5,22.));
#34054=CARTESIAN_POINT('',(25.45,-0.3,22.));
#34055=CARTESIAN_POINT('',(25.45,18.,22.));
#34056=CARTESIAN_POINT('',(34.7765679801409,-0.3,19.3142103002592));
#34057=CARTESIAN_POINT('Origin',(30.5,-0.3,22.));
#34058=CARTESIAN_POINT('Ctrl Pts',(34.7765679801409,-0.3,19.3142103002592));
#34059=CARTESIAN_POINT('Ctrl Pts',(34.9059508242202,-0.300000000000001,
19.5202258822768));
#34060=CARTESIAN_POINT('Ctrl Pts',(35.0195507283414,-0.34517160022148,19.7352882545191));
#34061=CARTESIAN_POINT('Ctrl Pts',(35.2238731819906,-0.522391523218817,
20.1939695646418));
#34062=CARTESIAN_POINT('Ctrl Pts',(35.3033062350033,-0.666213665915556,
20.42817906326));
#34063=CARTESIAN_POINT('Ctrl Pts',(35.3584694985011,-0.840438680575254,
20.6224009726343));
#34064=CARTESIAN_POINT('Ctrl Pts',(35.3590743849931,-0.842362231347438,
20.6245360702757));
#34065=CARTESIAN_POINT('Ctrl Pts',(35.3596764192561,-0.84428983422674,20.6266664279477));
#34066=CARTESIAN_POINT('',(30.7302400397221,1.5,27.0447487077266));
#34067=CARTESIAN_POINT('Origin',(30.5,1.5,22.));
#34068=CARTESIAN_POINT('',(30.7302400397217,-0.844289851346252,27.0447487077266));
#34069=CARTESIAN_POINT('',(30.7302400397221,-2.7,27.0447487077266));
#34070=CARTESIAN_POINT('',(29.3008405049219,-0.3,26.9055597545401));
#34071=CARTESIAN_POINT('Ctrl Pts',(30.7302400397215,-0.84428985134645,27.0447487077266));
#34072=CARTESIAN_POINT('Ctrl Pts',(30.7124846491452,-0.828813695351024,
27.0455590556881));
#34073=CARTESIAN_POINT('Ctrl Pts',(30.6944584562156,-0.813666012125142,
27.0462877270776));
#34074=CARTESIAN_POINT('Ctrl Pts',(30.4892675361419,-0.647229741839043,
27.0534512698364));
#34075=CARTESIAN_POINT('Ctrl Pts',(30.2640772634479,-0.51948243683466,27.0505384638851));
#34076=CARTESIAN_POINT('Ctrl Pts',(29.7858333404989,-0.346841431540347,
27.0046852545821));
#34077=CARTESIAN_POINT('Ctrl Pts',(29.5415138144396,-0.3,26.9643921200114));
#34078=CARTESIAN_POINT('Ctrl Pts',(29.3008405049219,-0.3,26.9055597545401));
#34079=CARTESIAN_POINT('Origin',(30.5,-0.3,22.));
#34080=CARTESIAN_POINT('Origin',(-35.5422371315094,-2.7,20.6547211791723));
#34081=CARTESIAN_POINT('',(-35.7247978384157,-1.8,20.6827759114759));
#34082=CARTESIAN_POINT('',(-35.3596764246031,-0.844289851346258,20.6266664468684));
#34083=CARTESIAN_POINT('Ctrl Pts',(-35.3596764246028,-0.844289851346478,
20.6266664468687));
#34084=CARTESIAN_POINT('Ctrl Pts',(-35.4623482961748,-0.961189991573225,
20.6424443868256));
#34085=CARTESIAN_POINT('Ctrl Pts',(-35.5522597002982,-1.105341946597,20.6562613818212));
#34086=CARTESIAN_POINT('Ctrl Pts',(-35.6808305167185,-1.40677945093785,
20.6760193017913));
#34087=CARTESIAN_POINT('Ctrl Pts',(-35.7247978384157,-1.61916866909503,
20.6827759114759));
#34088=CARTESIAN_POINT('Ctrl Pts',(-35.7247978384157,-1.8,20.6827759114759));
#34089=CARTESIAN_POINT('',(-35.3596764246032,1.5,20.6266664468687));
#34090=CARTESIAN_POINT('',(-35.3596764246032,-2.7,20.6266664468687));
#34091=CARTESIAN_POINT('',(-35.724797838416,0.551098954354631,20.6827759114753));
#34092=CARTESIAN_POINT('Ctrl Pts',(-35.7247978384164,0.55109895435502,20.682775911476));
#34093=CARTESIAN_POINT('Ctrl Pts',(-35.6230425085721,0.667215858413704,
20.6671388196416));
#34094=CARTESIAN_POINT('Ctrl Pts',(-35.5338848608002,0.809115390969431,
20.6534376569794));
#34095=CARTESIAN_POINT('Ctrl Pts',(-35.40452588567,1.10798634108372,20.6335586179471));
#34096=CARTESIAN_POINT('Ctrl Pts',(-35.3596764246032,1.31962574714054,20.6266664468687));
#34097=CARTESIAN_POINT('Ctrl Pts',(-35.3596764246032,1.5,20.6266664468687));
#34098=CARTESIAN_POINT('',(-35.7247978384157,-2.7,20.6827759114759));
#34099=CARTESIAN_POINT('Origin',(-30.5,18.,22.));
#34100=CARTESIAN_POINT('',(-35.55,17.5,22.));
#34101=CARTESIAN_POINT('Origin',(-30.5,17.5,22.));
#34102=CARTESIAN_POINT('',(-35.55,1.5,22.));
#34103=CARTESIAN_POINT('',(-35.55,18.,22.));
#34104=CARTESIAN_POINT('Origin',(-30.5,1.5,22.));
#34105=CARTESIAN_POINT('',(-34.7765679801409,-0.3,19.3142103002592));
#34106=CARTESIAN_POINT('Ctrl Pts',(-35.359676424603,-0.844289851346454,
20.6266664468682));
#34107=CARTESIAN_POINT('Ctrl Pts',(-35.3548608196211,-0.828871170093358,
20.609625952993));
#34108=CARTESIAN_POINT('Ctrl Pts',(-35.3498834808043,-0.813778557683737,
20.5923560119679));
#34109=CARTESIAN_POINT('Ctrl Pts',(-35.291962158532,-0.647352440369088,
20.3954487204406));
#34110=CARTESIAN_POINT('Ctrl Pts',(-35.2181442235994,-0.519566075661792,
20.1826589576689));
#34111=CARTESIAN_POINT('Ctrl Pts',(-35.0237121665274,-0.346861287281918,
19.7432418804637));
#34112=CARTESIAN_POINT('Ctrl Pts',(-34.9083644556171,-0.300000000000001,
19.5240690941071));
#34113=CARTESIAN_POINT('Ctrl Pts',(-34.7765679801409,-0.3,19.3142103002592));
#34114=CARTESIAN_POINT('',(-29.3008405049219,-0.3,26.9055597545401));
#34115=CARTESIAN_POINT('Origin',(-30.5,-0.3,22.));
#34116=CARTESIAN_POINT('',(-30.7302400262003,-0.844289827774839,27.0447487083437));
#34117=CARTESIAN_POINT('Ctrl Pts',(-29.3008405049219,-0.3,26.9055597545401));
#34118=CARTESIAN_POINT('Ctrl Pts',(-29.5371794327976,-0.3,26.9633325844718));
#34119=CARTESIAN_POINT('Ctrl Pts',(-29.7771237213194,-0.34518030422705,
27.0032706405318));
#34120=CARTESIAN_POINT('Ctrl Pts',(-30.2768601749874,-0.522423095905239,
27.0524182450713));
#34121=CARTESIAN_POINT('Ctrl Pts',(-30.52416303416,-0.666251438728489,27.0538881066326));
#34122=CARTESIAN_POINT('Ctrl Pts',(-30.7258446252404,-0.840467297370239,
27.0449478768001));
#34123=CARTESIAN_POINT('Ctrl Pts',(-30.7280449816332,-0.842376569836416,
27.0448488891723));
#34124=CARTESIAN_POINT('Ctrl Pts',(-30.7302400203693,-0.844289834478454,
27.0447487086098));
#34125=CARTESIAN_POINT('',(-30.7302400397221,1.5,27.0447487077266));
#34126=CARTESIAN_POINT('',(-30.7302400397221,-2.7,27.0447487077266));
#34127=CARTESIAN_POINT('Origin',(-30.5,1.5,22.));
#34128=CARTESIAN_POINT('Origin',(-30.8144664255862,-2.7,27.2091305669295));
#34129=CARTESIAN_POINT('',(-30.8986928114466,0.551098954346123,27.3735124261366));
#34130=CARTESIAN_POINT('Ctrl Pts',(-30.7302400397221,1.5,27.0447487077266));
#34131=CARTESIAN_POINT('Ctrl Pts',(-30.7302400397221,1.31962574714054,27.0447487077266));
#34132=CARTESIAN_POINT('Ctrl Pts',(-30.7509318308399,1.10798634108372,27.0851321939616));
#34133=CARTESIAN_POINT('Ctrl Pts',(-30.8106130138229,0.809115390967542,
27.2016099902902));
#34134=CARTESIAN_POINT('Ctrl Pts',(-30.8517468731915,0.667215858409751,
27.2818895868779));
#34135=CARTESIAN_POINT('Ctrl Pts',(-30.8986928114527,0.551098954350096,
27.3735124261369));
#34136=CARTESIAN_POINT('',(-30.8986928114504,-1.8,27.3735124261324));
#34137=CARTESIAN_POINT('Ctrl Pts',(-30.8986928114504,-1.8,27.3735124261324));
#34138=CARTESIAN_POINT('Ctrl Pts',(-30.8986928114504,-1.61916866909503,
27.3735124261324));
#34139=CARTESIAN_POINT('Ctrl Pts',(-30.8784080050129,-1.40677945093785,
27.333923238474));
#34140=CARTESIAN_POINT('Ctrl Pts',(-30.8190904464838,-1.10534194040792,
27.2181551159985));
#34141=CARTESIAN_POINT('Ctrl Pts',(-30.77760883065,-0.961189978595379,27.1371968145879));
#34142=CARTESIAN_POINT('Ctrl Pts',(-30.7302400332229,-0.844289835307704,
27.0447486950422));
#34143=CARTESIAN_POINT('',(-30.8986928114504,-2.7,27.3735124261324));
#34144=CARTESIAN_POINT('Origin',(30.8144664255862,-2.7,27.2091305669295));
#34145=CARTESIAN_POINT('',(30.8986928114504,-1.8,27.3735124261324));
#34146=CARTESIAN_POINT('Ctrl Pts',(30.7302400397219,-0.84428985134648,27.0447487077262));
#34147=CARTESIAN_POINT('Ctrl Pts',(30.7776088345681,-0.961189991573226,
27.1371968222349));
#34148=CARTESIAN_POINT('Ctrl Pts',(30.8190904477017,-1.105341946597,27.2181551183754));
#34149=CARTESIAN_POINT('Ctrl Pts',(30.8784080050129,-1.40677945093785,27.333923238474));
#34150=CARTESIAN_POINT('Ctrl Pts',(30.8986928114504,-1.61916866909503,27.3735124261324));
#34151=CARTESIAN_POINT('Ctrl Pts',(30.8986928114504,-1.8,27.3735124261324));
#34152=CARTESIAN_POINT('',(30.8986928114499,0.551098954354628,27.3735124261329));
#34153=CARTESIAN_POINT('Ctrl Pts',(30.8986928114507,0.551098954355018,27.373512426133));
#34154=CARTESIAN_POINT('Ctrl Pts',(30.8517468731903,0.667215858413702,27.2818895868756));
#34155=CARTESIAN_POINT('Ctrl Pts',(30.8106130138225,0.809115390969429,27.2016099902895));
#34156=CARTESIAN_POINT('Ctrl Pts',(30.7509318308399,1.10798634108372,27.0851321939616));
#34157=CARTESIAN_POINT('Ctrl Pts',(30.7302400397221,1.31962574714054,27.0447487077266));
#34158=CARTESIAN_POINT('Ctrl Pts',(30.7302400397221,1.5,27.0447487077266));
#34159=CARTESIAN_POINT('',(30.8986928114504,-2.7,27.3735124261324));
#34160=CARTESIAN_POINT('Origin',(30.5,17.75,-55.));
#34161=CARTESIAN_POINT('',(24.95,18.,-55.));
#34162=CARTESIAN_POINT('Origin',(30.5,18.,-55.));
#34163=CARTESIAN_POINT('',(25.2,17.75,-55.));
#34164=CARTESIAN_POINT('Origin',(0.,18.,-16.5));
#34165=CARTESIAN_POINT('',(38.,18.,-75.));
#34166=CARTESIAN_POINT('',(64.5,18.,-48.5));
#34167=CARTESIAN_POINT('Origin',(38.,18.,-48.5));
#34168=CARTESIAN_POINT('',(-38.,18.,-75.));
#34169=CARTESIAN_POINT('',(19.,18.,-75.));
#34170=CARTESIAN_POINT('',(-64.5,18.,-48.5));
#34171=CARTESIAN_POINT('Origin',(-38.,18.,-48.5));
#34172=CARTESIAN_POINT('',(-64.5,18.,15.5));
#34173=CARTESIAN_POINT('',(-64.5,18.,-32.5));
#34174=CARTESIAN_POINT('',(-38.,18.,42.));
#34175=CARTESIAN_POINT('Origin',(-38.,18.,15.5));
#34176=CARTESIAN_POINT('',(38.,18.,42.));
#34177=CARTESIAN_POINT('',(-19.,18.,42.));
#34178=CARTESIAN_POINT('',(64.5,18.,15.5));
#34179=CARTESIAN_POINT('Origin',(38.,18.,15.5));
#34180=CARTESIAN_POINT('',(64.5,18.,-0.500000000000003));
#34181=CARTESIAN_POINT('',(-36.05,18.,22.));
#34182=CARTESIAN_POINT('Origin',(-30.5,18.,22.));
#34183=CARTESIAN_POINT('',(-36.05,18.,-55.));
#34184=CARTESIAN_POINT('Origin',(-30.5,18.,-55.));
#34185=CARTESIAN_POINT('',(-59.2,18.,7.34788079488411E-16));
#34186=CARTESIAN_POINT('Origin',(-53.2,18.,0.));
#34187=CARTESIAN_POINT('',(26.05,18.,4.44089209850063E-15));
#34188=CARTESIAN_POINT('',(26.05,18.,-33.));
#34189=CARTESIAN_POINT('',(26.05,18.,-24.75));
#34190=CARTESIAN_POINT('',(-26.05,18.,0.));
#34191=CARTESIAN_POINT('Origin',(0.,18.,0.));
#34192=CARTESIAN_POINT('',(-26.05,18.,-33.));
#34193=CARTESIAN_POINT('',(-26.05,18.,-8.25));
#34194=CARTESIAN_POINT('Origin',(0.,18.,-33.));
#34195=CARTESIAN_POINT('',(26.49,18.,-16.5));
#34196=CARTESIAN_POINT('Origin',(30.5,18.,-16.5));
#34197=CARTESIAN_POINT('',(-34.51,18.,-16.5));
#34198=CARTESIAN_POINT('Origin',(-30.5,18.,-16.5));
#34199=CARTESIAN_POINT('',(47.2,18.,7.34788079488411E-16));
#34200=CARTESIAN_POINT('Origin',(53.2,18.,0.));
#34201=CARTESIAN_POINT('',(24.95,18.,22.));
#34202=CARTESIAN_POINT('Origin',(30.5,18.,22.));
#34203=CARTESIAN_POINT('Origin',(-30.5,17.75,22.));
#34204=CARTESIAN_POINT('',(-35.8,17.75,22.));
#34205=CARTESIAN_POINT('Origin',(30.5,17.75,22.));
#34206=CARTESIAN_POINT('',(25.2,17.75,22.));
#34207=CARTESIAN_POINT('Origin',(-30.5,17.75,-55.));
#34208=CARTESIAN_POINT('',(-35.8,17.75,-55.));
#34209=CARTESIAN_POINT('Origin',(53.2,17.75,0.));
#34210=CARTESIAN_POINT('',(47.7,17.5,-6.73555739531044E-16));
#34211=CARTESIAN_POINT('',(47.45,17.75,7.04171909509728E-16));
#34212=CARTESIAN_POINT('Origin',(53.2,17.5,0.));
#34213=CARTESIAN_POINT('Origin',(53.2,-0.1,0.));
#34214=CARTESIAN_POINT('',(47.7,0.5,6.73555739531044E-16));
#34215=CARTESIAN_POINT('Origin',(53.2,0.5,0.));
#34216=CARTESIAN_POINT('',(47.7,-0.1,6.73555739531044E-16));
#34217=CARTESIAN_POINT('Origin',(-53.2,17.75,0.));
#34218=CARTESIAN_POINT('',(-58.7,17.5,-6.73555739531044E-16));
#34219=CARTESIAN_POINT('',(-58.95,17.75,7.04171909509728E-16));
#34220=CARTESIAN_POINT('Origin',(-53.2,17.5,0.));
#34221=CARTESIAN_POINT('Origin',(-53.2,-0.1,0.));
#34222=CARTESIAN_POINT('',(-58.7,0.5,6.73555739531044E-16));
#34223=CARTESIAN_POINT('Origin',(-53.2,0.5,0.));
#34224=CARTESIAN_POINT('',(-58.7,-0.1,6.73555739531044E-16));
#34225=CARTESIAN_POINT('Ctrl Pts',(-46.2750334800828,0.00185294611160958,
-44.0483053101957));
#34226=CARTESIAN_POINT('Ctrl Pts',(-46.2692140102843,0.00164657951619625,
-44.0483519609257));
#34227=CARTESIAN_POINT('Ctrl Pts',(-46.2265311890134,0.000220053554164141,
-44.0487734988259));
#34228=CARTESIAN_POINT('Ctrl Pts',(-46.1797598454879,1.29647441628285E-5,
-44.0493466615837));
#34229=CARTESIAN_POINT('Ctrl Pts',(-46.1722185099715,-1.25208261182028E-17,
-44.0494259364697));
#34230=CARTESIAN_POINT('Ctrl Pts',(-46.1707625875413,0.,-44.0494422439817));
#34231=CARTESIAN_POINT('Ctrl Pts',(-46.2750334800828,0.00185294611160958,
-44.3812532465669));
#34232=CARTESIAN_POINT('Ctrl Pts',(-46.2692140102843,0.0016465795161962,
-44.3812687968102));
#34233=CARTESIAN_POINT('Ctrl Pts',(-46.2265311890134,0.000220053554164124,
-44.3813630297282));
#34234=CARTESIAN_POINT('Ctrl Pts',(-46.1797598454879,1.29647441628394E-5,
-44.3816138834835));
#34235=CARTESIAN_POINT('Ctrl Pts',(-46.1722185099715,-7.54565250469149E-18,
-44.3816267886582));
#34236=CARTESIAN_POINT('Ctrl Pts',(-46.1707625875413,0.,-44.3816322244955));
#34237=CARTESIAN_POINT('Ctrl Pts',(-46.2750334800828,0.00185294611160958,
-44.7142011829381));
#34238=CARTESIAN_POINT('Ctrl Pts',(-46.2692140102843,0.00164657951619616,
-44.7141856326948));
#34239=CARTESIAN_POINT('Ctrl Pts',(-46.2264061493503,-2.42006109810558E-5,
-44.7139663601137));
#34240=CARTESIAN_POINT('Ctrl Pts',(-46.1797424783604,0.000164604021204162,
-44.7138231788941));
#34241=CARTESIAN_POINT('Ctrl Pts',(-46.1722185099715,-2.56641760752889E-18,
-44.7138276408467));
#34242=CARTESIAN_POINT('Ctrl Pts',(-46.1707625875413,0.,-44.7138222050094));
#34243=CARTESIAN_POINT('Ctrl Pts',(-46.2750334800828,0.00185294611160958,
-45.0471491193093));
#34244=CARTESIAN_POINT('Ctrl Pts',(-46.2692140102843,0.00164657951619612,
-45.0471024685793));
#34245=CARTESIAN_POINT('Ctrl Pts',(-46.2265311890134,0.000220053554162325,
-45.0466809306791));
#34246=CARTESIAN_POINT('Ctrl Pts',(-46.1797598454878,1.29647441628376E-5,
-45.0461077679213));
#34247=CARTESIAN_POINT('Ctrl Pts',(-46.1722185099715,2.40785117657972E-18,
-45.0460284930352));
#34248=CARTESIAN_POINT('Ctrl Pts',(-46.1707625875413,0.,-45.0460121855233));
#34249=CARTESIAN_POINT('',(-46.2750334800828,0.00185294611160958,-44.0483053101957));
#34250=CARTESIAN_POINT('Ctrl Pts',(-46.1707625875413,-2.22044604925031E-16,
-44.0494422439817));
#34251=CARTESIAN_POINT('Ctrl Pts',(-46.1712260120785,-2.29034413256906E-16,
-44.0494370532511));
#34252=CARTESIAN_POINT('Ctrl Pts',(-46.1716940067242,9.12216844862265E-8,
-44.0494318096041));
#34253=CARTESIAN_POINT('Ctrl Pts',(-46.1722703781186,3.87472611551587E-7,
-44.0494252934764));
#34254=CARTESIAN_POINT('Ctrl Pts',(-46.1728752899714,6.98393137625681E-7,
-44.0494184546864));
#34255=CARTESIAN_POINT('Ctrl Pts',(-46.1735992866602,1.23194503986655E-6,
-44.0494102174312));
#34256=CARTESIAN_POINT('Ctrl Pts',(-46.1745042934384,2.38657547613208E-6,
-44.0493998460925));
#34257=CARTESIAN_POINT('Ctrl Pts',(-46.1754684855519,3.61671605358732E-6,
-44.0493887964925));
#34258=CARTESIAN_POINT('Ctrl Pts',(-46.1766377387174,5.55516755122873E-6,
-44.0493753288015));
#34259=CARTESIAN_POINT('Ctrl Pts',(-46.1780277790772,8.99934440856676E-6,
-44.0493592449597));
#34260=CARTESIAN_POINT('Ctrl Pts',(-46.1795622676003,1.28014281552638E-5,
-44.0493414897409));
#34261=CARTESIAN_POINT('Ctrl Pts',(-46.1813652342406,1.84658046869166E-5,
-44.0493205524466));
#34262=CARTESIAN_POINT('Ctrl Pts',(-46.183395156043,2.72127176232928E-5,
-44.0492969087164));
#34263=CARTESIAN_POINT('Ctrl Pts',(-46.1859419093286,3.81866523005328E-5,
-44.0492672451365));
#34264=CARTESIAN_POINT('Ctrl Pts',(-46.1888446371058,5.41281456188157E-5,
-44.049233333982));
#34265=CARTESIAN_POINT('Ctrl Pts',(-46.1919381576189,7.64762491831661E-5,
-44.0491971278456));
#34266=CARTESIAN_POINT('Ctrl Pts',(-46.1952200088624,0.000100184885075284,
-44.0491587175124));
#34267=CARTESIAN_POINT('Ctrl Pts',(-46.198709812785,0.000131146817816346,
-44.0491178019999));
#34268=CARTESIAN_POINT('Ctrl Pts',(-46.2021957015517,0.000168532538723509,
-44.0490769551091));
#34269=CARTESIAN_POINT('Ctrl Pts',(-46.2048367108624,0.000196857033166613,
-44.0490460083331));
#34270=CARTESIAN_POINT('Ctrl Pts',(-46.207474324971,0.000228767928640852,
-44.0490151153336));
#34271=CARTESIAN_POINT('Ctrl Pts',(-46.2100500271557,0.000263295917068085,
-44.0489850380078));
#34272=CARTESIAN_POINT('Ctrl Pts',(-46.2123742451676,0.000294452691750434,
-44.0489578973459));
#34273=CARTESIAN_POINT('Ctrl Pts',(-46.2146474763278,0.000327690884695818,
-44.0489314272062));
#34274=CARTESIAN_POINT('Ctrl Pts',(-46.2168680460012,0.000362622665149637,
-44.0489057363541));
#34275=CARTESIAN_POINT('Ctrl Pts',(-46.2190586240439,0.000397082647276686,
-44.0488803924898));
#34276=CARTESIAN_POINT('Ctrl Pts',(-46.2211970152928,0.000433137034800887,
-44.0488558169149));
#34277=CARTESIAN_POINT('Ctrl Pts',(-46.2233355230111,0.00047149090490195,
-44.0488315276206));
#34278=CARTESIAN_POINT('Ctrl Pts',(-46.2254211663469,0.000508896658874311,
-44.048807838763));
#34279=CARTESIAN_POINT('Ctrl Pts',(-46.2275162736585,0.000548663598881684,
-44.048784324577));
#34280=CARTESIAN_POINT('Ctrl Pts',(-46.229662604295,0.000591779397137282,
-44.0487605858922));
#34281=CARTESIAN_POINT('Ctrl Pts',(-46.2319694831195,0.000638120310465147,
-44.0487350715244));
#34282=CARTESIAN_POINT('Ctrl Pts',(-46.2343350335908,0.000688360290181702,
-44.0487093036337));
#34283=CARTESIAN_POINT('Ctrl Pts',(-46.2367509866092,0.000742716673596044,
-44.0486833825405));
#34284=CARTESIAN_POINT('Ctrl Pts',(-46.2395110312765,0.000804814754574078,
-44.0486537696405));
#34285=CARTESIAN_POINT('Ctrl Pts',(-46.2423361082531,0.000872336312489005,
-44.0486239662077));
#34286=CARTESIAN_POINT('Ctrl Pts',(-46.2451470433618,0.000943604228376804,
-44.0485947611566));
#34287=CARTESIAN_POINT('Ctrl Pts',(-46.2490414567667,0.00104234244759405,
-44.0485542989836));
#34288=CARTESIAN_POINT('Ctrl Pts',(-46.2529045939084,0.00114840209597425,
-44.0485150363574));
#34289=CARTESIAN_POINT('Ctrl Pts',(-46.2564328497428,0.00125139174850086,
-44.0484798418561));
#34290=CARTESIAN_POINT('Ctrl Pts',(-46.2590790416185,0.00132863398789582,
-44.0484534459802));
#34291=CARTESIAN_POINT('Ctrl Pts',(-46.261533087147,0.00140389724199395,
-44.0484293702208));
#34292=CARTESIAN_POINT('Ctrl Pts',(-46.2636886623346,0.00147212889993908,
-44.0484085450809));
#34293=CARTESIAN_POINT('Ctrl Pts',(-46.2654946449701,0.00152929470429269,
-44.0483910973753));
#34294=CARTESIAN_POINT('Ctrl Pts',(-46.267090598365,0.00158146111034102,
-44.0483759344752));
#34295=CARTESIAN_POINT('Ctrl Pts',(-46.2684508145559,0.00162671007904525,
-44.0483632289425));
#34296=CARTESIAN_POINT('Ctrl Pts',(-46.2697296616146,0.00166925222118772,
-44.048351283464));
#34297=CARTESIAN_POINT('Ctrl Pts',(-46.2707995465537,0.00170564250685707,
-44.048341514987));
#34298=CARTESIAN_POINT('Ctrl Pts',(-46.2716824580706,0.0017359725457522,
-44.0483336475365));
#34299=CARTESIAN_POINT('Ctrl Pts',(-46.2725053682963,0.0017642414024576,
-44.0483263147457));
#34300=CARTESIAN_POINT('Ctrl Pts',(-46.273165643982,0.00178723762246348,
-44.0483206352252));
#34301=CARTESIAN_POINT('Ctrl Pts',(-46.2737251009273,0.00180683428706385,
-44.0483159663184));
#34302=CARTESIAN_POINT('Ctrl Pts',(-46.2742130349626,0.00182392564631187,
-44.0483118943007));
#34303=CARTESIAN_POINT('Ctrl Pts',(-46.2746246568584,0.00183844866426981,
-44.0483085874533));
#34304=CARTESIAN_POINT('Ctrl Pts',(-46.2750334800827,0.00185294611160836,
-44.0483053101957));
#34305=CARTESIAN_POINT('',(-46.2750334800828,0.00185294611160958,-45.0471491193093));
#34306=CARTESIAN_POINT('Ctrl Pts',(-46.2750334800828,0.00185294611160958,
-45.0471491193093));
#34307=CARTESIAN_POINT('Ctrl Pts',(-46.2750334800828,0.00185294611160958,
-44.7142011829381));
#34308=CARTESIAN_POINT('Ctrl Pts',(-46.2750334800828,0.00185294611160958,
-44.3812532465669));
#34309=CARTESIAN_POINT('Ctrl Pts',(-46.2750334800828,0.00185294611160958,
-44.0483053101957));
#34310=CARTESIAN_POINT('Ctrl Pts',(-46.2750334800828,0.00185294611160991,
-45.0471491193093));
#34311=CARTESIAN_POINT('Ctrl Pts',(-46.2745703659484,0.00183652343213913,
-45.0471454068384));
#34312=CARTESIAN_POINT('Ctrl Pts',(-46.2741026813164,0.00182002913551302,
-45.0471416470788));
#34313=CARTESIAN_POINT('Ctrl Pts',(-46.2735266846993,0.00179989061882035,
-45.0471368004589));
#34314=CARTESIAN_POINT('Ctrl Pts',(-46.272922163659,0.00177875480534642,
-45.0471317138253));
#34315=CARTESIAN_POINT('Ctrl Pts',(-46.2721986280875,0.00175361200744172,
-45.0471254328191));
#34316=CARTESIAN_POINT('Ctrl Pts',(-46.2712941819279,0.00172265954511253,
-45.0471173077251));
#34317=CARTESIAN_POINT('Ctrl Pts',(-46.2703305802151,0.00168968262836036,
-45.047108651207));
#34318=CARTESIAN_POINT('Ctrl Pts',(-46.2691620271534,0.00165012867729241,
-45.0470979049924));
#34319=CARTESIAN_POINT('Ctrl Pts',(-46.2677727834885,0.00160423233980689,
-45.0470848469776));
#34320=CARTESIAN_POINT('Ctrl Pts',(-46.2662391395715,0.00155356546215624,
-45.0470704316916));
#34321=CARTESIAN_POINT('Ctrl Pts',(-46.2644371217823,0.001495217018528,
-45.0470532033005));
#34322=CARTESIAN_POINT('Ctrl Pts',(-46.2624081930856,0.00143187557828095,
-45.0470334723104));
#34323=CARTESIAN_POINT('Ctrl Pts',(-46.2598623899414,0.00135239775434378,
-45.0470087148033));
#34324=CARTESIAN_POINT('Ctrl Pts',(-46.2569605947754,0.00126521876820982,
-45.0469800244132));
#34325=CARTESIAN_POINT('Ctrl Pts',(-46.2538679066071,0.00117763891592237,
-45.0469488787412));
#34326=CARTESIAN_POINT('Ctrl Pts',(-46.2505882042891,0.00108476312989613,
-45.0469158496975));
#34327=CARTESIAN_POINT('Ctrl Pts',(-46.2471005941737,0.000991719524369893,
-45.0468801237951));
#34328=CARTESIAN_POINT('Ctrl Pts',(-46.2436166498116,0.000905201076382811,
-45.0468437234767));
#34329=CARTESIAN_POINT('Ctrl Pts',(-46.2409766290361,0.0008396401843567,
-45.0468161404883));
#34330=CARTESIAN_POINT('Ctrl Pts',(-46.2383398635848,0.000777766532132296,
-45.0467881851458));
#34331=CARTESIAN_POINT('Ctrl Pts',(-46.2357648305552,0.00072069456144308,
-45.0467604449209));
#34332=CARTESIAN_POINT('Ctrl Pts',(-46.2334411807933,0.00066919414588216,
-45.0467354127887));
#34333=CARTESIAN_POINT('Ctrl Pts',(-46.2311683745646,0.000621574660653182,
-45.0467105626822));
#34334=CARTESIAN_POINT('Ctrl Pts',(-46.2289480715865,0.000577512604324371,
-45.0466859283192));
#34335=CARTESIAN_POINT('Ctrl Pts',(-46.2267571009757,0.000534032650722002,
-45.0466616194001));
#34336=CARTESIAN_POINT('Ctrl Pts',(-46.2246181983236,0.000493996445433125,
-45.0466375306524));
#34337=CARTESIAN_POINT('Ctrl Pts',(-46.2224789858344,0.000456253937658024,
-45.0466131580609));
#34338=CARTESIAN_POINT('Ctrl Pts',(-46.2203933191886,0.000419456148754817,
-45.0465893955308));
#34339=CARTESIAN_POINT('Ctrl Pts',(-46.2182980063535,0.000384680303810759,
-45.0465652657332));
#34340=CARTESIAN_POINT('Ctrl Pts',(-46.2161513192572,0.000351435419324808,
-45.0465403951498));
#34341=CARTESIAN_POINT('Ctrl Pts',(-46.2138440203937,0.000315703204635488,
-45.0465136637883));
#34342=CARTESIAN_POINT('Ctrl Pts',(-46.2114778723633,0.000281787957705771,
-45.0464860818021));
#34343=CARTESIAN_POINT('Ctrl Pts',(-46.2090611791439,0.000250206967382205,
-45.0464578399095));
#34344=CARTESIAN_POINT('Ctrl Pts',(-46.2063001182845,0.000214125831560948,
-45.0464255736774));
#34345=CARTESIAN_POINT('Ctrl Pts',(-46.2034738288062,0.00018116946976453,
-45.046392454497));
#34346=CARTESIAN_POINT('Ctrl Pts',(-46.2006615752144,0.000152480845408531,
-45.0463594963285));
#34347=CARTESIAN_POINT('Ctrl Pts',(-46.1967660663297,0.000112741615848296,
-45.046313842964));
#34348=CARTESIAN_POINT('Ctrl Pts',(-46.1929016183748,8.14691463179917E-5,
-45.0462685501633));
#34349=CARTESIAN_POINT('Ctrl Pts',(-46.1893720134758,5.90616066560301E-5,
-45.0462272825148));
#34350=CARTESIAN_POINT('Ctrl Pts',(-46.1867248098016,4.22559519095589E-5,
-45.0461963317784));
#34351=CARTESIAN_POINT('Ctrl Pts',(-46.1842697342872,3.03183594517789E-5,
-45.0461676865023));
#34352=CARTESIAN_POINT('Ctrl Pts',(-46.1821131987253,2.19691435525693E-5,
-45.0461425976401));
#34353=CARTESIAN_POINT('Ctrl Pts',(-46.1803063686599,1.49738430462828E-5,
-45.0461215772074));
#34354=CARTESIAN_POINT('Ctrl Pts',(-46.1787096280764,1.04521897691233E-5,
-45.0461030584842));
#34355=CARTESIAN_POINT('Ctrl Pts',(-46.1773487225908,7.39546431272053E-6,
-45.0460873323693));
#34356=CARTESIAN_POINT('Ctrl Pts',(-46.1760692107157,4.52155678447191E-6,
-45.0460725468084));
#34357=CARTESIAN_POINT('Ctrl Pts',(-46.1749987537671,2.92603171308054E-6,
-45.0460602361923));
#34358=CARTESIAN_POINT('Ctrl Pts',(-46.1741153616204,1.91616332645417E-6,
-45.0460501300432));
#34359=CARTESIAN_POINT('Ctrl Pts',(-46.1732919932801,9.74912421790196E-7,
-45.0460407105763));
#34360=CARTESIAN_POINT('Ctrl Pts',(-46.1726313429966,5.41797940506856E-7,
-45.0460332083471));
#34361=CARTESIAN_POINT('Ctrl Pts',(-46.172071556338,2.9201856199812E-7,
-45.0460268901009));
#34362=CARTESIAN_POINT('Ctrl Pts',(-46.171583423441,7.42114211156187E-8,
-45.0460213806022));
#34363=CARTESIAN_POINT('Ctrl Pts',(-46.1711716076359,-2.2137356598813E-16,
-45.0460167668801));
#34364=CARTESIAN_POINT('Ctrl Pts',(-46.1707625875413,-2.22044604925031E-16,
-45.0460121855233));
#34365=CARTESIAN_POINT('Ctrl Pts',(-46.2750334800828,0.00185294611160958,
-45.0471491193093));
#34366=CARTESIAN_POINT('Ctrl Pts',(-46.814203289689,0.0209726669473543,
-45.0514712768415));
#34367=CARTESIAN_POINT('Ctrl Pts',(-47.6898108873463,0.308848973617175,
-45.0129318213479));
#34368=CARTESIAN_POINT('Ctrl Pts',(-48.346446182696,0.985587673094209,-44.9222599738363));
#34369=CARTESIAN_POINT('Ctrl Pts',(-48.4368145112785,1.33275179473165,-44.9012806053457));
#34370=CARTESIAN_POINT('Ctrl Pts',(-48.4368145112785,1.50000000000004,-44.9012806053457));
#34371=CARTESIAN_POINT('Ctrl Pts',(-46.2750334800828,0.00185294611160958,
-44.7142011829381));
#34372=CARTESIAN_POINT('Ctrl Pts',(-46.814203289689,0.0209726669473542,
-44.7156419021155));
#34373=CARTESIAN_POINT('Ctrl Pts',(-47.6898108873463,0.308848973617175,
-44.702795416951));
#34374=CARTESIAN_POINT('Ctrl Pts',(-48.346446182696,0.985587673094209,-44.6725714677804));
#34375=CARTESIAN_POINT('Ctrl Pts',(-48.4368145112785,1.33275179473165,-44.6655783449502));
#34376=CARTESIAN_POINT('Ctrl Pts',(-48.4368145112785,1.50000000000004,-44.6655783449502));
#34377=CARTESIAN_POINT('Ctrl Pts',(-46.2750334800828,0.00185294611160958,
-44.3812532465669));
#34378=CARTESIAN_POINT('Ctrl Pts',(-46.814203289689,0.0209726669473541,
-44.3798125273895));
#34379=CARTESIAN_POINT('Ctrl Pts',(-47.6898108873463,0.308848973617173,
-44.392659012554));
#34380=CARTESIAN_POINT('Ctrl Pts',(-48.346446182696,0.985587673094209,-44.4228829617245));
#34381=CARTESIAN_POINT('Ctrl Pts',(-48.4368145112785,1.33275179473165,-44.4298760845547));
#34382=CARTESIAN_POINT('Ctrl Pts',(-48.4368145112785,1.50000000000003,-44.4298760845547));
#34383=CARTESIAN_POINT('Ctrl Pts',(-46.2750334800828,0.00185294611160958,
-44.0483053101957));
#34384=CARTESIAN_POINT('Ctrl Pts',(-46.814203289689,0.020972666947354,-44.0439831526635));
#34385=CARTESIAN_POINT('Ctrl Pts',(-47.6898108873463,0.308848973617173,
-44.0825226081571));
#34386=CARTESIAN_POINT('Ctrl Pts',(-48.346446182696,0.985587673094209,-44.1731944556686));
#34387=CARTESIAN_POINT('Ctrl Pts',(-48.4368145112785,1.33275179473165,-44.1941738241592));
#34388=CARTESIAN_POINT('Ctrl Pts',(-48.4368145112785,1.50000000000003,-44.1941738241592));
#34389=CARTESIAN_POINT('',(-48.4368145112785,1.50000000000002,-44.1941738241592));
#34390=CARTESIAN_POINT('Ctrl Pts',(-46.2750334800828,0.00185294611160958,
-44.0483053101957));
#34391=CARTESIAN_POINT('Ctrl Pts',(-46.814203289689,0.020972666947354,-44.0439831526635));
#34392=CARTESIAN_POINT('Ctrl Pts',(-47.6898108873463,0.308848973617173,
-44.0825226081571));
#34393=CARTESIAN_POINT('Ctrl Pts',(-48.346446182696,0.985587673094209,-44.1731944556686));
#34394=CARTESIAN_POINT('Ctrl Pts',(-48.4368145112785,1.33275179473165,-44.1941738241592));
#34395=CARTESIAN_POINT('Ctrl Pts',(-48.4368145112785,1.50000000000003,-44.1941738241592));
#34396=CARTESIAN_POINT('',(-48.4368145112785,1.50000000000002,-44.9012806053457));
#34397=CARTESIAN_POINT('',(-48.4368145112785,1.50000000000002,-44.1941738241592));
#34398=CARTESIAN_POINT('Ctrl Pts',(-48.4368145112785,1.50000000000004,-44.9012806053457));
#34399=CARTESIAN_POINT('Ctrl Pts',(-48.4368145112785,1.33275179473165,-44.9012806053457));
#34400=CARTESIAN_POINT('Ctrl Pts',(-48.346446182696,0.985587673094209,-44.9222599738363));
#34401=CARTESIAN_POINT('Ctrl Pts',(-47.6898108873463,0.308848973617175,
-45.0129318213479));
#34402=CARTESIAN_POINT('Ctrl Pts',(-46.814203289689,0.0209726669473543,
-45.0514712768415));
#34403=CARTESIAN_POINT('Ctrl Pts',(-46.2750334800828,0.00185294611160958,
-45.0471491193093));
#34404=CARTESIAN_POINT('Origin',(-48.4368145112785,4.,-44.5477272147525));
#34405=CARTESIAN_POINT('',(-48.4368145112785,4.,-44.1941738241592));
#34406=CARTESIAN_POINT('',(-48.4368145112785,4.,-44.9012806053458));
#34407=CARTESIAN_POINT('',(-48.4368145112785,4.,-30.5238636073762));
#34408=CARTESIAN_POINT('',(-48.4368145112785,4.,-44.9012806053458));
#34409=CARTESIAN_POINT('',(-48.4368145112785,4.,-44.1941738241592));
#34410=CARTESIAN_POINT('Origin',(-42.5440475583121,1.5,-48.6727272147525));
#34411=CARTESIAN_POINT('',(-44.9012806053458,1.5,-48.4368145112785));
#34412=CARTESIAN_POINT('',(-43.6047077300919,1.5,-49.7333873865323));
#34413=CARTESIAN_POINT('',(-45.0471491193093,0.00185294611161013,-46.2750334800827));
#34414=CARTESIAN_POINT('Ctrl Pts',(-45.0471491193093,0.00185294611161013,
-46.2750334800827));
#34415=CARTESIAN_POINT('Ctrl Pts',(-45.0514712768415,0.0209726669473565,
-46.8142032896889));
#34416=CARTESIAN_POINT('Ctrl Pts',(-45.0129318213479,0.308848973617163,
-47.6898108873462));
#34417=CARTESIAN_POINT('Ctrl Pts',(-44.9222599738363,0.985587673094179,
-48.3464461826959));
#34418=CARTESIAN_POINT('Ctrl Pts',(-44.9012806053458,1.33275179473162,-48.4368145112785));
#34419=CARTESIAN_POINT('Ctrl Pts',(-44.9012806053458,1.5,-48.4368145112785));
#34420=CARTESIAN_POINT('Ctrl Pts',(-45.0460121855233,-2.22044604925031E-16,
-46.1707625875413));
#34421=CARTESIAN_POINT('Ctrl Pts',(-45.0460173762539,-2.21088104837496E-16,
-46.1712260120786));
#34422=CARTESIAN_POINT('Ctrl Pts',(-45.0460226199009,9.12216842420496E-8,
-46.1716940067243));
#34423=CARTESIAN_POINT('Ctrl Pts',(-45.0460291360286,3.87472611329542E-7,
-46.1722703781187));
#34424=CARTESIAN_POINT('Ctrl Pts',(-45.0460359748186,6.98393137422036E-7,
-46.1728752899715));
#34425=CARTESIAN_POINT('Ctrl Pts',(-45.0460442120738,1.23194503982883E-6,
-46.1735992866603));
#34426=CARTESIAN_POINT('Ctrl Pts',(-45.0460545834124,2.38657547613208E-6,
-46.1745042934385));
#34427=CARTESIAN_POINT('Ctrl Pts',(-45.0460656330125,3.61671605361644E-6,
-46.175468485552));
#34428=CARTESIAN_POINT('Ctrl Pts',(-45.0460791007035,5.55516755121E-6,-46.1766377387174));
#34429=CARTESIAN_POINT('Ctrl Pts',(-45.0460951845453,8.99934440856676E-6,
-46.1780277790772));
#34430=CARTESIAN_POINT('Ctrl Pts',(-45.0461129397641,1.2801428155372E-5,
-46.1795622676004));
#34431=CARTESIAN_POINT('Ctrl Pts',(-45.0461338770584,1.84658046875068E-5,
-46.1813652342407));
#34432=CARTESIAN_POINT('Ctrl Pts',(-45.0461575207886,2.7212717624181E-5,
-46.1833951560432));
#34433=CARTESIAN_POINT('Ctrl Pts',(-45.0461871843685,3.81866523016351E-5,
-46.1859419093288));
#34434=CARTESIAN_POINT('Ctrl Pts',(-45.046221095523,5.41281456200928E-5,
-46.188844637106));
#34435=CARTESIAN_POINT('Ctrl Pts',(-45.0462573016594,7.64762491847204E-5,
-46.1919381576191));
#34436=CARTESIAN_POINT('Ctrl Pts',(-45.0462957119926,0.000100184885075293,
-46.1952200088624));
#34437=CARTESIAN_POINT('Ctrl Pts',(-45.0463366275051,0.000131146817813724,
-46.1987098127846));
#34438=CARTESIAN_POINT('Ctrl Pts',(-45.0463774743959,0.000168532538717292,
-46.2021957015511));
#34439=CARTESIAN_POINT('Ctrl Pts',(-45.0464084211719,0.000196857033159762,
-46.2048367108618));
#34440=CARTESIAN_POINT('Ctrl Pts',(-45.0464393141714,0.000228767928633612,
-46.2074743249703));
#34441=CARTESIAN_POINT('Ctrl Pts',(-45.0464693914972,0.000263295917060313,
-46.210050027155));
#34442=CARTESIAN_POINT('Ctrl Pts',(-45.0464965321591,0.000294452691741994,
-46.2123742451669));
#34443=CARTESIAN_POINT('Ctrl Pts',(-45.0465230022988,0.000327690884686502,
-46.2146474763272));
#34444=CARTESIAN_POINT('Ctrl Pts',(-45.0465486931509,0.000362622665139645,
-46.2168680460005));
#34445=CARTESIAN_POINT('Ctrl Pts',(-45.0465740370152,0.000397082647263859,
-46.2190586240431));
#34446=CARTESIAN_POINT('Ctrl Pts',(-45.0465986125901,0.000433137034784962,
-46.2211970152918));
#34447=CARTESIAN_POINT('Ctrl Pts',(-45.0466229018844,0.00047149090488241,
-46.22333552301));
#34448=CARTESIAN_POINT('Ctrl Pts',(-45.046646590742,0.000508896658854249,
-46.2254211663458));
#34449=CARTESIAN_POINT('Ctrl Pts',(-45.046670104928,0.00054866359886092,
-46.2275162736575));
#34450=CARTESIAN_POINT('Ctrl Pts',(-45.0466938436128,0.000591779397115744,
-46.2296626042939));
#34451=CARTESIAN_POINT('Ctrl Pts',(-45.0467193579806,0.00063812031043945,
-46.2319694831182));
#34452=CARTESIAN_POINT('Ctrl Pts',(-45.0467451258713,0.000688360290151415,
-46.2343350335893));
#34453=CARTESIAN_POINT('Ctrl Pts',(-45.0467710469645,0.000742716673560517,
-46.2367509866076));
#34454=CARTESIAN_POINT('Ctrl Pts',(-45.0468006598645,0.000804814754530438,
-46.2395110312746));
#34455=CARTESIAN_POINT('Ctrl Pts',(-45.0468304632973,0.00087233631243586,
-46.2423361082509));
#34456=CARTESIAN_POINT('Ctrl Pts',(-45.0468596683484,0.000943604228314632,
-46.2451470433594));
#34457=CARTESIAN_POINT('Ctrl Pts',(-45.0469001305214,0.00104234244753431,
-46.2490414567645));
#34458=CARTESIAN_POINT('Ctrl Pts',(-45.0469393931475,0.0011484020959196,
-46.2529045939064));
#34459=CARTESIAN_POINT('Ctrl Pts',(-45.0469745876488,0.0012513917484529,
-46.2564328497411));
#34460=CARTESIAN_POINT('Ctrl Pts',(-45.0470009835248,0.00132863398785288,
-46.2590790416171));
#34461=CARTESIAN_POINT('Ctrl Pts',(-45.0470250592842,0.00140389724195716,
-46.2615330871458));
#34462=CARTESIAN_POINT('Ctrl Pts',(-45.0470458844242,0.00147212889990822,
-46.2636886623335));
#34463=CARTESIAN_POINT('Ctrl Pts',(-45.0470633321297,0.00152929470426462,
-46.2654946449692));
#34464=CARTESIAN_POINT('Ctrl Pts',(-45.0470784950298,0.00158146111031593,
-46.2670905983642));
#34465=CARTESIAN_POINT('Ctrl Pts',(-45.0470912005626,0.00162671007902326,
-46.2684508145552));
#34466=CARTESIAN_POINT('Ctrl Pts',(-45.047103146041,0.00166925222116762,
-46.269729661614));
#34467=CARTESIAN_POINT('Ctrl Pts',(-45.047112914518,0.00170564250683925,
-46.2707995465531));
#34468=CARTESIAN_POINT('Ctrl Pts',(-45.0471207819685,0.00173597254573643,
-46.2716824580701));
#34469=CARTESIAN_POINT('Ctrl Pts',(-45.0471281147594,0.00176424140244397,
-46.2725053682959));
#34470=CARTESIAN_POINT('Ctrl Pts',(-45.0471337942798,0.00178723762245191,
-46.2731656439817));
#34471=CARTESIAN_POINT('Ctrl Pts',(-45.0471384631867,0.00180683428705364,
-46.273725100927));
#34472=CARTESIAN_POINT('Ctrl Pts',(-45.0471425352043,0.00182392564630702,
-46.2742130349624));
#34473=CARTESIAN_POINT('Ctrl Pts',(-45.0471458420517,0.00183844866426805,
-46.2746246568583));
#34474=CARTESIAN_POINT('Ctrl Pts',(-45.0471491193093,0.00185294611161013,
-46.2750334800828));
#34475=CARTESIAN_POINT('Origin',(-48.7903679018718,4.,-44.5477272147525));
#34476=CARTESIAN_POINT('',(-44.9012806053458,4.,-48.4368145112785));
#34477=CARTESIAN_POINT('',(-43.6047077300919,4.,-49.7333873865323));
#34478=CARTESIAN_POINT('',(-44.9012806053458,4.,-48.4368145112785));
#34479=CARTESIAN_POINT('Ctrl Pts',(-45.0471491193093,0.00185294611161013,
-46.2750334800827));
#34480=CARTESIAN_POINT('Ctrl Pts',(-45.0471024685793,0.00164657951619665,
-46.2692140102843));
#34481=CARTESIAN_POINT('Ctrl Pts',(-45.0466809306791,0.000220053554162977,
-46.2265311890134));
#34482=CARTESIAN_POINT('Ctrl Pts',(-45.0461077679213,1.29647441628623E-5,
-46.1797598454878));
#34483=CARTESIAN_POINT('Ctrl Pts',(-45.0460284930352,2.98573545895863E-18,
-46.1722185099715));
#34484=CARTESIAN_POINT('Ctrl Pts',(-45.0460121855233,0.,-46.1707625875413));
#34485=CARTESIAN_POINT('Ctrl Pts',(-44.7142011829381,0.00185294611161013,
-46.2750334800827));
#34486=CARTESIAN_POINT('Ctrl Pts',(-44.7141856326948,0.00164657951619654,
-46.2692140102843));
#34487=CARTESIAN_POINT('Ctrl Pts',(-44.7140913997768,0.00022005355416289,
-46.2265311890134));
#34488=CARTESIAN_POINT('Ctrl Pts',(-44.7138405460215,1.29647441628478E-5,
-46.1797598454878));
#34489=CARTESIAN_POINT('Ctrl Pts',(-44.7138276408467,2.02507727125502E-18,
-46.1722185099715));
#34490=CARTESIAN_POINT('Ctrl Pts',(-44.7138222050094,0.,-46.1707625875413));
#34491=CARTESIAN_POINT('Ctrl Pts',(-44.3812532465669,0.00185294611161013,
-46.2750334800828));
#34492=CARTESIAN_POINT('Ctrl Pts',(-44.3812687968102,0.0016465795161965,
-46.2692140102843));
#34493=CARTESIAN_POINT('Ctrl Pts',(-44.3814880693913,-2.42006109825039E-5,
-46.2264061493503));
#34494=CARTESIAN_POINT('Ctrl Pts',(-44.3816312506108,0.00016460402120339,
-46.1797424783604));
#34495=CARTESIAN_POINT('Ctrl Pts',(-44.3816267886582,1.05075738695553E-18,
-46.1722185099715));
#34496=CARTESIAN_POINT('Ctrl Pts',(-44.3816322244956,0.,-46.1707625875413));
#34497=CARTESIAN_POINT('Ctrl Pts',(-44.0483053101957,0.00185294611161013,
-46.2750334800828));
#34498=CARTESIAN_POINT('Ctrl Pts',(-44.0483519609257,0.00164657951619639,
-46.2692140102843));
#34499=CARTESIAN_POINT('Ctrl Pts',(-44.0487734988259,0.000220053554162283,
-46.2265311890134));
#34500=CARTESIAN_POINT('Ctrl Pts',(-44.0493466615837,1.29647441628678E-5,
-46.1797598454878));
#34501=CARTESIAN_POINT('Ctrl Pts',(-44.0494259364698,9.6314047063189E-20,
-46.1722185099715));
#34502=CARTESIAN_POINT('Ctrl Pts',(-44.0494422439817,0.,-46.1707625875413));
#34503=CARTESIAN_POINT('',(-44.0483053101957,0.00185294611161013,-46.2750334800828));
#34504=CARTESIAN_POINT('Ctrl Pts',(-44.0483053101957,0.00185294611161013,
-46.2750334800828));
#34505=CARTESIAN_POINT('Ctrl Pts',(-44.3812532465669,0.00185294611161013,
-46.2750334800828));
#34506=CARTESIAN_POINT('Ctrl Pts',(-44.7142011829381,0.00185294611161013,
-46.2750334800827));
#34507=CARTESIAN_POINT('Ctrl Pts',(-45.0471491193093,0.00185294611161013,
-46.2750334800827));
#34508=CARTESIAN_POINT('Ctrl Pts',(-44.0483053101957,0.00185294611161058,
-46.2750334800828));
#34509=CARTESIAN_POINT('Ctrl Pts',(-44.0483090226666,0.00183652343213972,
-46.2745703659484));
#34510=CARTESIAN_POINT('Ctrl Pts',(-44.0483127824262,0.0018200291355136,
-46.2741026813164));
#34511=CARTESIAN_POINT('Ctrl Pts',(-44.0483176290461,0.0017998906188208,
-46.2735266846993));
#34512=CARTESIAN_POINT('Ctrl Pts',(-44.0483227156797,0.00177875480534672,
-46.272922163659));
#34513=CARTESIAN_POINT('Ctrl Pts',(-44.0483289966859,0.00175361200744154,
-46.2721986280875));
#34514=CARTESIAN_POINT('Ctrl Pts',(-44.0483371217799,0.00172265954511208,
-46.2712941819278));
#34515=CARTESIAN_POINT('Ctrl Pts',(-44.048345778298,0.00168968262836068,
-46.2703305802151));
#34516=CARTESIAN_POINT('Ctrl Pts',(-44.0483565245126,0.00165012867729383,
-46.2691620271535));
#34517=CARTESIAN_POINT('Ctrl Pts',(-44.0483695825273,0.00160423233980977,
-46.2677727834886));
#34518=CARTESIAN_POINT('Ctrl Pts',(-44.0483839978134,0.00155356546215882,
-46.2662391395715));
#34519=CARTESIAN_POINT('Ctrl Pts',(-44.0484012262045,0.0014952170185302,
-46.2644371217823));
#34520=CARTESIAN_POINT('Ctrl Pts',(-44.0484209571946,0.0014318755782825,
-46.2624081930856));
#34521=CARTESIAN_POINT('Ctrl Pts',(-44.0484457147017,0.00135239775434602,
-46.2598623899414));
#34522=CARTESIAN_POINT('Ctrl Pts',(-44.0484744050917,0.00126521876821268,
-46.2569605947755));
#34523=CARTESIAN_POINT('Ctrl Pts',(-44.0485055507637,0.00117763891592593,
-46.2538679066073));
#34524=CARTESIAN_POINT('Ctrl Pts',(-44.0485385798074,0.00108476312989682,
-46.2505882042891));
#34525=CARTESIAN_POINT('Ctrl Pts',(-44.0485743057099,0.000991719524367669,
-46.2471005941736));
#34526=CARTESIAN_POINT('Ctrl Pts',(-44.0486107060283,0.000905201076378148,
-46.2436166498114));
#34527=CARTESIAN_POINT('Ctrl Pts',(-44.0486382890167,0.000839640184351458,
-46.2409766290359));
#34528=CARTESIAN_POINT('Ctrl Pts',(-44.0486662443592,0.000777766532126836,
-46.2383398635846));
#34529=CARTESIAN_POINT('Ctrl Pts',(-44.0486939845841,0.000720694561437307,
-46.2357648305549));
#34530=CARTESIAN_POINT('Ctrl Pts',(-44.0487190167163,0.000669194145876824,
-46.233441180793));
#34531=CARTESIAN_POINT('Ctrl Pts',(-44.0487438668228,0.000621574660648363,
-46.2311683745643));
#34532=CARTESIAN_POINT('Ctrl Pts',(-44.0487685011858,0.00057751260431993,
-46.2289480715863));
#34533=CARTESIAN_POINT('Ctrl Pts',(-44.0487928101048,0.000534032650715443,
-46.2267571009754));
#34534=CARTESIAN_POINT('Ctrl Pts',(-44.0488168988526,0.00049399644542456,
-46.2246181983231));
#34535=CARTESIAN_POINT('Ctrl Pts',(-44.0488412714441,0.00045625393764781,
-46.2224789858338));
#34536=CARTESIAN_POINT('Ctrl Pts',(-44.0488650339742,0.000419456148745576,
-46.220393319188));
#34537=CARTESIAN_POINT('Ctrl Pts',(-44.0488891637718,0.00038468030380222,
-46.218298006353));
#34538=CARTESIAN_POINT('Ctrl Pts',(-44.0489140343552,0.000351435419317037,
-46.2161513192567));
#34539=CARTESIAN_POINT('Ctrl Pts',(-44.0489407657167,0.00031570320462769,
-46.2138440203931));
#34540=CARTESIAN_POINT('Ctrl Pts',(-44.0489683477029,0.000281787957698108,
-46.2114778723627));
#34541=CARTESIAN_POINT('Ctrl Pts',(-44.0489965895955,0.000250206967374655,
-46.2090611791433));
#34542=CARTESIAN_POINT('Ctrl Pts',(-44.0490288558276,0.000214125831553833,
-46.2063001182839));
#34543=CARTESIAN_POINT('Ctrl Pts',(-44.049061975008,0.000181169469757948,
-46.2034738288056));
#34544=CARTESIAN_POINT('Ctrl Pts',(-44.0490949331765,0.000152480845402536,
-46.2006615752138));
#34545=CARTESIAN_POINT('Ctrl Pts',(-44.049140586541,0.000112741615843626,
-46.1967660663292));
#34546=CARTESIAN_POINT('Ctrl Pts',(-44.0491858793417,8.14691463146172E-5,
-46.1929016183743));
#34547=CARTESIAN_POINT('Ctrl Pts',(-44.0492271469902,5.90616066535876E-5,
-46.1893720134754));
#34548=CARTESIAN_POINT('Ctrl Pts',(-44.0492580977266,4.22559519078155E-5,
-46.1867248098013));
#34549=CARTESIAN_POINT('Ctrl Pts',(-44.0492867430027,3.03183594507372E-5,
-46.1842697342869));
#34550=CARTESIAN_POINT('Ctrl Pts',(-44.0493118318649,2.19691435519032E-5,
-46.182113198725));
#34551=CARTESIAN_POINT('Ctrl Pts',(-44.0493328522976,1.49738430459103E-5,
-46.1803063686597));
#34552=CARTESIAN_POINT('Ctrl Pts',(-44.0493513710208,1.04521897685428E-5,
-46.1787096280762));
#34553=CARTESIAN_POINT('Ctrl Pts',(-44.0493670971357,7.39546431227645E-6,
-46.1773487225907));
#34554=CARTESIAN_POINT('Ctrl Pts',(-44.0493818826966,4.52155678414927E-6,
-46.1760692107156));
#34555=CARTESIAN_POINT('Ctrl Pts',(-44.0493941933127,2.92603171325643E-6,
-46.174998753767));
#34556=CARTESIAN_POINT('Ctrl Pts',(-44.0494042994618,1.91616332667621E-6,
-46.1741153616203));
#34557=CARTESIAN_POINT('Ctrl Pts',(-44.0494137189287,9.74912422044362E-7,
-46.17329199328));
#34558=CARTESIAN_POINT('Ctrl Pts',(-44.0494212211579,5.41797940269787E-7,
-46.1726313429966));
#34559=CARTESIAN_POINT('Ctrl Pts',(-44.0494275394041,2.92018561776075E-7,
-46.1720715563379));
#34560=CARTESIAN_POINT('Ctrl Pts',(-44.0494330489028,7.4211420916902E-8,
-46.171583423441));
#34561=CARTESIAN_POINT('Ctrl Pts',(-44.0494376626249,-2.22022958507713E-16,
-46.1711716076359));
#34562=CARTESIAN_POINT('Ctrl Pts',(-44.0494422439817,-2.22044604925031E-16,
-46.1707625875413));
#34563=CARTESIAN_POINT('Ctrl Pts',(-44.0483053101957,0.00185294611161013,
-46.2750334800828));
#34564=CARTESIAN_POINT('Ctrl Pts',(-44.0439831526635,0.020972666947357,
-46.814203289689));
#34565=CARTESIAN_POINT('Ctrl Pts',(-44.0825226081571,0.308848973617166,
-47.6898108873462));
#34566=CARTESIAN_POINT('Ctrl Pts',(-44.1731944556687,0.985587673094177,
-48.3464461826959));
#34567=CARTESIAN_POINT('Ctrl Pts',(-44.1941738241592,1.33275179473161,-48.4368145112785));
#34568=CARTESIAN_POINT('Ctrl Pts',(-44.1941738241592,1.5,-48.4368145112785));
#34569=CARTESIAN_POINT('Ctrl Pts',(-44.3812532465669,0.00185294611161013,
-46.2750334800828));
#34570=CARTESIAN_POINT('Ctrl Pts',(-44.3798125273895,0.0209726669473568,
-46.814203289689));
#34571=CARTESIAN_POINT('Ctrl Pts',(-44.392659012554,0.308848973617166,-47.6898108873462));
#34572=CARTESIAN_POINT('Ctrl Pts',(-44.4228829617246,0.985587673094178,
-48.3464461826959));
#34573=CARTESIAN_POINT('Ctrl Pts',(-44.4298760845547,1.33275179473162,-48.4368145112785));
#34574=CARTESIAN_POINT('Ctrl Pts',(-44.4298760845547,1.5,-48.4368145112785));
#34575=CARTESIAN_POINT('Ctrl Pts',(-44.7142011829381,0.00185294611161013,
-46.2750334800827));
#34576=CARTESIAN_POINT('Ctrl Pts',(-44.7156419021155,0.0209726669473567,
-46.8142032896889));
#34577=CARTESIAN_POINT('Ctrl Pts',(-44.7027954169509,0.308848973617164,
-47.6898108873462));
#34578=CARTESIAN_POINT('Ctrl Pts',(-44.6725714677804,0.985587673094178,
-48.3464461826959));
#34579=CARTESIAN_POINT('Ctrl Pts',(-44.6655783449502,1.33275179473162,-48.4368145112785));
#34580=CARTESIAN_POINT('Ctrl Pts',(-44.6655783449502,1.5,-48.4368145112785));
#34581=CARTESIAN_POINT('Ctrl Pts',(-45.0471491193093,0.00185294611161013,
-46.2750334800827));
#34582=CARTESIAN_POINT('Ctrl Pts',(-45.0514712768415,0.0209726669473565,
-46.8142032896889));
#34583=CARTESIAN_POINT('Ctrl Pts',(-45.0129318213479,0.308848973617163,
-47.6898108873462));
#34584=CARTESIAN_POINT('Ctrl Pts',(-44.9222599738363,0.985587673094179,
-48.3464461826959));
#34585=CARTESIAN_POINT('Ctrl Pts',(-44.9012806053458,1.33275179473162,-48.4368145112785));
#34586=CARTESIAN_POINT('Ctrl Pts',(-44.9012806053458,1.5,-48.4368145112785));
#34587=CARTESIAN_POINT('',(-44.1941738241592,1.5,-48.4368145112785));
#34588=CARTESIAN_POINT('',(-44.9012806053458,1.5,-48.4368145112785));
#34589=CARTESIAN_POINT('Ctrl Pts',(-44.1941738241592,1.5,-48.4368145112785));
#34590=CARTESIAN_POINT('Ctrl Pts',(-44.1941738241592,1.33275179473161,-48.4368145112785));
#34591=CARTESIAN_POINT('Ctrl Pts',(-44.1731944556687,0.985587673094177,
-48.3464461826959));
#34592=CARTESIAN_POINT('Ctrl Pts',(-44.0825226081571,0.308848973617166,
-47.6898108873462));
#34593=CARTESIAN_POINT('Ctrl Pts',(-44.0439831526635,0.020972666947357,
-46.814203289689));
#34594=CARTESIAN_POINT('Ctrl Pts',(-44.0483053101957,0.00185294611161013,
-46.2750334800828));
#34595=CARTESIAN_POINT('Origin',(-44.5477272147525,4.,-48.4368145112785));
#34596=CARTESIAN_POINT('',(-44.1941738241592,4.,-48.4368145112785));
#34597=CARTESIAN_POINT('',(-22.2738636073762,4.,-48.4368145112785));
#34598=CARTESIAN_POINT('',(-44.1941738241592,4.,-48.4368145112785));
#34599=CARTESIAN_POINT('Origin',(-26.3988636073762,1.5,-28.5201839509359));
#34600=CARTESIAN_POINT('',(-31.0449275599944,1.5,-35.2875682471136));
#34601=CARTESIAN_POINT('',(-25.3382034355964,1.5,-29.5808441227157));
#34602=CARTESIAN_POINT('Ctrl Pts',(-31.0952102098472,0.,-33.2165305534069));
#34603=CARTESIAN_POINT('Ctrl Pts',(-31.0951683510534,1.11734401589392E-19,
-33.2190692967299));
#34604=CARTESIAN_POINT('Ctrl Pts',(-31.0951264183426,3.32975363939714E-6,
-33.2216080407998));
#34605=CARTESIAN_POINT('Ctrl Pts',(-31.0915543966548,0.000569671234466166,
-33.4374895579288));
#34606=CARTESIAN_POINT('Ctrl Pts',(-31.0874717825085,0.024650660129702,
-33.6519250591448));
#34607=CARTESIAN_POINT('Ctrl Pts',(-31.0788092838543,0.119724494999934,
-34.0573511387189));
#34608=CARTESIAN_POINT('Ctrl Pts',(-31.0742145020816,0.188992076600158,
-34.2510845845319));
#34609=CARTESIAN_POINT('Ctrl Pts',(-31.0647171688648,0.382511576258832,
-34.6214706148708));
#34610=CARTESIAN_POINT('Ctrl Pts',(-31.0597601262273,0.510857073213101,
-34.7982799030232));
#34611=CARTESIAN_POINT('Ctrl Pts',(-31.0522501584557,0.790024881159197,
-35.0535067624131));
#34612=CARTESIAN_POINT('Ctrl Pts',(-31.0494412598632,0.927714535375556,
-35.1443641805612));
#34613=CARTESIAN_POINT('Ctrl Pts',(-31.0458492854634,1.2139998648115,-35.2589537310755));
#34614=CARTESIAN_POINT('Ctrl Pts',(-31.0449275599944,1.35542940125327,-35.2875682471136));
#34615=CARTESIAN_POINT('Ctrl Pts',(-31.0449275599944,1.5,-35.2875682471136));
#34616=CARTESIAN_POINT('Origin',(-44.5477272147525,4.,-48.7903679018718));
#34617=CARTESIAN_POINT('',(-31.0449275599944,4.,-35.2875682471136));
#34618=CARTESIAN_POINT('',(-25.3382034355964,4.,-29.5808441227157));
#34619=CARTESIAN_POINT('',(-31.0449275599944,4.,-35.2875682471136));
#34620=CARTESIAN_POINT('Origin',(-53.2,0.25,0.));
#34621=CARTESIAN_POINT('',(-58.95,0.25,-7.04171909509728E-16));
#34622=CARTESIAN_POINT('Origin',(53.2,0.25,0.));
#34623=CARTESIAN_POINT('',(47.45,0.25,-7.04171909509728E-16));
#34624=CARTESIAN_POINT('Origin',(44.5477272147525,4.,-48.4368145112785));
#34625=CARTESIAN_POINT('',(44.1941738241592,4.,-48.4368145112785));
#34626=CARTESIAN_POINT('',(44.9012806053458,4.,-48.4368145112785));
#34627=CARTESIAN_POINT('',(22.2738636073762,4.,-48.4368145112785));
#34628=CARTESIAN_POINT('',(44.9012806053458,1.5,-48.4368145112785));
#34629=CARTESIAN_POINT('',(44.9012806053458,4.,-48.4368145112785));
#34630=CARTESIAN_POINT('',(44.1941738241592,1.5,-48.4368145112785));
#34631=CARTESIAN_POINT('',(44.9012806053458,1.5,-48.4368145112785));
#34632=CARTESIAN_POINT('',(44.1941738241592,4.,-48.4368145112785));
#34633=CARTESIAN_POINT('Origin',(45.4316106912357,1.5,-47.5529310347953));
#34634=CARTESIAN_POINT('',(45.6083873865323,0.500000000000005,-47.729707730092));
#34635=CARTESIAN_POINT('',(45.6083873865323,0.500000000000005,-47.729707730092));
#34636=CARTESIAN_POINT('Origin',(45.2548339959391,1.5,-47.3761543394987));
#34637=CARTESIAN_POINT('Origin',(45.6083873865323,1.5,-47.729707730092));
#34638=CARTESIAN_POINT('Origin',(41.3066106912357,0.25,-51.6779310347953));
#34639=CARTESIAN_POINT('',(47.729707730092,0.5,-45.6083873865323));
#34640=CARTESIAN_POINT('',(47.729707730092,0.5,-45.6083873865323));
#34641=CARTESIAN_POINT('',(41.4833873865323,0.5,-51.854707730092));
#34642=CARTESIAN_POINT('Origin',(47.5529310347953,1.5,-45.4316106912357));
#34643=CARTESIAN_POINT('',(48.4368145112785,1.5,-44.9012806053458));
#34644=CARTESIAN_POINT('',(48.4368145112785,1.5,-44.1941738241592));
#34645=CARTESIAN_POINT('',(48.4368145112785,1.5,-44.9012806053458));
#34646=CARTESIAN_POINT('Origin',(47.3761543394987,1.5,-45.254833995939));
#34647=CARTESIAN_POINT('Origin',(47.729707730092,1.5,-45.6083873865323));
#34648=CARTESIAN_POINT('Origin',(48.4368145112785,4.,-44.5477272147525));
#34649=CARTESIAN_POINT('',(48.4368145112785,4.,-44.9012806053458));
#34650=CARTESIAN_POINT('',(48.4368145112785,4.,-44.1941738241592));
#34651=CARTESIAN_POINT('',(48.4368145112785,4.,-30.5238636073763));
#34652=CARTESIAN_POINT('',(48.4368145112785,4.,-44.1941738241592));
#34653=CARTESIAN_POINT('',(48.4368145112785,4.,-44.9012806053458));
#34654=CARTESIAN_POINT('Origin',(44.5477272147525,4.,-48.7903679018718));
#34655=CARTESIAN_POINT('',(41.4833873865323,4.,-51.854707730092));
#34656=CARTESIAN_POINT('Origin',(0.,2.5,0.));
#34657=CARTESIAN_POINT('',(-13.3416640641263,4.,43.5));
#34658=CARTESIAN_POINT('',(-17.7974717305577,2.5,43.5));
#34659=CARTESIAN_POINT('Ctrl Pts',(-17.7974717305577,2.5,43.5));
#34660=CARTESIAN_POINT('Ctrl Pts',(-17.7974717305577,2.55909958962217,43.5));
#34661=CARTESIAN_POINT('Ctrl Pts',(-17.7856223944691,2.62902218815019,43.5));
#34662=CARTESIAN_POINT('Ctrl Pts',(-17.7453636557976,2.75139686483799,43.5));
#34663=CARTESIAN_POINT('Ctrl Pts',(-17.706168118457,2.82532121452828,43.5));
#34664=CARTESIAN_POINT('Ctrl Pts',(-17.5359812657224,3.06819459814041,43.5));
#34665=CARTESIAN_POINT('Ctrl Pts',(-17.3144913010137,3.22642942545082,43.5));
#34666=CARTESIAN_POINT('Ctrl Pts',(-16.5770721718092,3.62923551489079,43.5));
#34667=CARTESIAN_POINT('Ctrl Pts',(-15.9375248631358,3.77596647975076,43.5));
#34668=CARTESIAN_POINT('Ctrl Pts',(-14.6274773462457,3.96791177668935,43.5));
#34669=CARTESIAN_POINT('Ctrl Pts',(-13.9550874901819,4.,43.5));
#34670=CARTESIAN_POINT('Ctrl Pts',(-13.3416640641263,4.,43.5));
#34671=CARTESIAN_POINT('',(17.7974717305577,2.5,43.5));
#34672=CARTESIAN_POINT('Origin',(0.,2.5,0.));
#34673=CARTESIAN_POINT('',(13.3416640641263,4.,43.5));
#34674=CARTESIAN_POINT('Ctrl Pts',(13.3416640641263,4.,43.5));
#34675=CARTESIAN_POINT('Ctrl Pts',(13.9550874901819,4.,43.5));
#34676=CARTESIAN_POINT('Ctrl Pts',(14.6274773462457,3.96791177668935,43.5));
#34677=CARTESIAN_POINT('Ctrl Pts',(15.9375248631358,3.77596647975076,43.5));
#34678=CARTESIAN_POINT('Ctrl Pts',(16.5770721718093,3.62923551489079,43.5));
#34679=CARTESIAN_POINT('Ctrl Pts',(17.3144913010137,3.22642942545082,43.5));
#34680=CARTESIAN_POINT('Ctrl Pts',(17.5359812657224,3.06819459814041,43.5));
#34681=CARTESIAN_POINT('Ctrl Pts',(17.706168118457,2.82532121452828,43.5));
#34682=CARTESIAN_POINT('Ctrl Pts',(17.7453636557976,2.75139686483799,43.5));
#34683=CARTESIAN_POINT('Ctrl Pts',(17.7856223944691,2.62902218815019,43.5));
#34684=CARTESIAN_POINT('Ctrl Pts',(17.7974717305577,2.55909958962217,43.5));
#34685=CARTESIAN_POINT('Ctrl Pts',(17.7974717305577,2.5,43.5));
#34686=CARTESIAN_POINT('Origin',(0.,4.,0.));
#34687=CARTESIAN_POINT('Origin',(0.,4.,0.));
#34688=CARTESIAN_POINT('',(-17.7974717305577,1.5,43.5));
#34689=CARTESIAN_POINT('',(-17.7974717305577,4.,43.5));
#34690=CARTESIAN_POINT('',(17.7974717305577,1.5,43.5));
#34691=CARTESIAN_POINT('Origin',(0.,1.5,0.));
#34692=CARTESIAN_POINT('',(17.7974717305577,4.,43.5));
#34693=CARTESIAN_POINT('Origin',(-53.2,1.5,0.));
#34694=CARTESIAN_POINT('',(-46.2240601503759,1.5,8.50507279301165));
#34695=CARTESIAN_POINT('Ctrl Pts',(-45.209022556391,0.,5.13753632549025));
#34696=CARTESIAN_POINT('Ctrl Pts',(-45.2101706901705,-1.40306832022943E-18,
5.14245954784658));
#34697=CARTESIAN_POINT('Ctrl Pts',(-45.2113202904355,2.87874308356214E-6,
5.1473824373595));
#34698=CARTESIAN_POINT('Ctrl Pts',(-45.3805806089602,0.000852747696532382,
5.87122802959633));
#34699=CARTESIAN_POINT('Ctrl Pts',(-45.5407068125259,0.0644575560773281,
6.42770684158595));
#34700=CARTESIAN_POINT('Ctrl Pts',(-45.7992896021911,0.262676028338797,
7.27728490933266));
#34701=CARTESIAN_POINT('Ctrl Pts',(-45.9058399421765,0.391768785578365,
7.59761029794946));
#34702=CARTESIAN_POINT('Ctrl Pts',(-46.0437392091658,0.637700968927193,
8.00108322240395));
#34703=CARTESIAN_POINT('Ctrl Pts',(-46.095986299131,0.7544352578638,8.14964878644437));
#34704=CARTESIAN_POINT('Ctrl Pts',(-46.165500553065,0.987918955923497,8.34412682404574));
#34705=CARTESIAN_POINT('Ctrl Pts',(-46.1888166753861,1.09129381988889,8.40843236441884));
#34706=CARTESIAN_POINT('Ctrl Pts',(-46.2170785613611,1.29969233992949,8.48604609926929));
#34707=CARTESIAN_POINT('Ctrl Pts',(-46.2240601503759,1.39848091468836,8.50507279301165));
#34708=CARTESIAN_POINT('Ctrl Pts',(-46.2240601503759,1.5,8.50507279301165));
#34709=CARTESIAN_POINT('',(-58.,1.5,9.8974744253269));
#34710=CARTESIAN_POINT('Origin',(-53.2,1.5,0.));
#34711=CARTESIAN_POINT('Ctrl Pts',(-59.5,0.,7.11055553385247));
#34712=CARTESIAN_POINT('Ctrl Pts',(-59.4982621111229,-1.43714039392157E-18,
7.11441720740624));
#34713=CARTESIAN_POINT('Ctrl Pts',(-59.4965230425191,3.02025636744488E-6,
7.11827835650607));
#34714=CARTESIAN_POINT('Ctrl Pts',(-59.2998658347014,0.000687024107797437,
7.5545495242394));
#34715=CARTESIAN_POINT('Ctrl Pts',(-59.0848279111169,0.0390861404131355,
7.99027457435746));
#34716=CARTESIAN_POINT('Ctrl Pts',(-58.6790205873,0.227280698650663,8.75389357006342));
#34717=CARTESIAN_POINT('Ctrl Pts',(-58.5106474320197,0.353869330585226,
9.04860693524616));
#34718=CARTESIAN_POINT('Ctrl Pts',(-58.2889293801926,0.605541836240553,
9.4260831564163));
#34719=CARTESIAN_POINT('Ctrl Pts',(-58.2055841166437,0.725339698576898,
9.56428617469307));
#34720=CARTESIAN_POINT('Ctrl Pts',(-58.0942335303233,0.966223567273987,
9.74614959515893));
#34721=CARTESIAN_POINT('Ctrl Pts',(-58.0567637695508,1.07370986494963,9.80652098494185));
#34722=CARTESIAN_POINT('Ctrl Pts',(-58.01124521301,1.29080573116058,9.87956234691206));
#34723=CARTESIAN_POINT('Ctrl Pts',(-58.,1.3939909411326,9.89747442532689));
#34724=CARTESIAN_POINT('Ctrl Pts',(-58.,1.5,9.89747442532689));
#34725=CARTESIAN_POINT('Origin',(0.,1.5,0.));
#34726=CARTESIAN_POINT('',(-30.8017856625229,1.5,35.5));
#34727=CARTESIAN_POINT('Ctrl Pts',(-26.4811253537307,0.,37.));
#34728=CARTESIAN_POINT('Ctrl Pts',(-26.4867878946248,1.06044817773062E-17,
36.9981824187244));
#34729=CARTESIAN_POINT('Ctrl Pts',(-26.4924502779527,3.30360139702406E-6,
36.9963643050345));
#34730=CARTESIAN_POINT('Ctrl Pts',(-27.6012019204162,0.00129824004375969,
36.6402452052783));
#34731=CARTESIAN_POINT('Ctrl Pts',(-28.6022785210026,0.127864463880204,
36.2954324644459));
#34732=CARTESIAN_POINT('Ctrl Pts',(-29.7527298503777,0.479548357456909,
35.8858963683834));
#34733=CARTESIAN_POINT('Ctrl Pts',(-30.0640351469117,0.619696008492602,
35.7724767899835));
#34734=CARTESIAN_POINT('Ctrl Pts',(-30.4199450706296,0.856752956966091,
35.6417681188669));
#34735=CARTESIAN_POINT('Ctrl Pts',(-30.5405284008673,0.955292659882126,
35.5971805278559));
#34736=CARTESIAN_POINT('Ctrl Pts',(-30.6877287941394,1.1384738095481,35.5425226152298));
#34737=CARTESIAN_POINT('Ctrl Pts',(-30.7342206529605,1.21379195435448,35.525203642034));
#34738=CARTESIAN_POINT('Ctrl Pts',(-30.7885863901991,1.36171319479544,35.5049304586301));
#34739=CARTESIAN_POINT('Ctrl Pts',(-30.8017856625229,1.42978275763033,35.5));
#34740=CARTESIAN_POINT('Ctrl Pts',(-30.8017856625229,1.5,35.5));
#34741=CARTESIAN_POINT('Origin',(0.,1.5,0.));
#34742=CARTESIAN_POINT('Origin',(-36.,1.5,13.5));
#34743=CARTESIAN_POINT('',(-58.,1.5,13.5));
#34744=CARTESIAN_POINT('Origin',(-59.5,1.5,13.5));
#34745=CARTESIAN_POINT('',(-36.,1.5,35.5));
#34746=CARTESIAN_POINT('Origin',(-36.,1.5,13.5));
#34747=CARTESIAN_POINT('Origin',(-36.,1.5,37.));
#34748=CARTESIAN_POINT('Origin',(-18.,1.5,37.));
#34749=CARTESIAN_POINT('',(-18.,1.5,35.5));
#34750=CARTESIAN_POINT('Origin',(-59.5,1.5,-31.5));
#34751=CARTESIAN_POINT('',(-58.,1.5,-31.5));
#34752=CARTESIAN_POINT('Origin',(0.,4.,0.));
#34753=CARTESIAN_POINT('',(-30.8017856625229,4.,35.5));
#34754=CARTESIAN_POINT('',(-30.8017856625229,4.,35.5));
#34755=CARTESIAN_POINT('',(-46.2240601503759,4.,8.50507279301165));
#34756=CARTESIAN_POINT('Origin',(0.,4.,0.));
#34757=CARTESIAN_POINT('',(-46.2240601503759,4.,8.50507279301165));
#34758=CARTESIAN_POINT('Origin',(-36.,0.,35.5));
#34759=CARTESIAN_POINT('',(-36.,4.,35.5));
#34760=CARTESIAN_POINT('',(-36.,0.,35.5));
#34761=CARTESIAN_POINT('',(36.,4.,35.5));
#34762=CARTESIAN_POINT('Origin',(-36.,0.,13.5));
#34763=CARTESIAN_POINT('',(-58.,4.,13.5));
#34764=CARTESIAN_POINT('',(-58.,0.,13.5));
#34765=CARTESIAN_POINT('Origin',(-36.,4.,13.5));
#34766=CARTESIAN_POINT('Origin',(0.,1.5,0.));
#34767=CARTESIAN_POINT('',(46.2240601503759,1.5,8.50507279301165));
#34768=CARTESIAN_POINT('Ctrl Pts',(45.209022556391,0.,5.1375363254903));
#34769=CARTESIAN_POINT('Ctrl Pts',(45.2102521007232,1.11258750894249E-19,
5.14280863804894));
#34770=CARTESIAN_POINT('Ctrl Pts',(45.2114833270665,3.30146167889055E-6,
5.14808056967696));
#34771=CARTESIAN_POINT('Ctrl Pts',(45.3784738591765,0.000901308928852578,
5.86208365506188));
#34772=CARTESIAN_POINT('Ctrl Pts',(45.5364437851314,0.0627444670134214,
6.4126471717855));
#34773=CARTESIAN_POINT('Ctrl Pts',(45.7956313154401,0.258490073791997,7.2662018107722));
#34774=CARTESIAN_POINT('Ctrl Pts',(45.9037816258573,0.388566620441501,7.59150909299489));
#34775=CARTESIAN_POINT('Ctrl Pts',(46.043055046971,0.636193465569317,7.99912982559317));
#34776=CARTESIAN_POINT('Ctrl Pts',(46.0956128185241,0.753321114945002,8.14859884634578));
#34777=CARTESIAN_POINT('Ctrl Pts',(46.1654106238969,0.987526374219774,8.34387849941688));
#34778=CARTESIAN_POINT('Ctrl Pts',(46.1887788399396,1.09104391483163,8.40832834536188));
#34779=CARTESIAN_POINT('Ctrl Pts',(46.2170749275856,1.29964148682512,8.48603621443855));
#34780=CARTESIAN_POINT('Ctrl Pts',(46.2240601503759,1.39845449738161,8.50507279301165));
#34781=CARTESIAN_POINT('Ctrl Pts',(46.2240601503759,1.5,8.50507279301165));
#34782=CARTESIAN_POINT('',(30.8017856625229,1.5,35.5));
#34783=CARTESIAN_POINT('Origin',(0.,1.5,0.));
#34784=CARTESIAN_POINT('Ctrl Pts',(26.4811253537307,0.,37.));
#34785=CARTESIAN_POINT('Ctrl Pts',(26.4867878946292,1.11294754654022E-19,
36.998182418723));
#34786=CARTESIAN_POINT('Ctrl Pts',(26.4924502779482,3.30360139191886E-6,
36.996364305036));
#34787=CARTESIAN_POINT('Ctrl Pts',(27.6012019219699,0.00129824004556856,
36.6402452047772));
#34788=CARTESIAN_POINT('Ctrl Pts',(28.6022785220106,0.127864464188313,36.2954324640871));
#34789=CARTESIAN_POINT('Ctrl Pts',(29.7527298503796,0.479548357457492,35.8858963683827));
#34790=CARTESIAN_POINT('Ctrl Pts',(30.0640351469129,0.619696008493419,35.7724767899831));
#34791=CARTESIAN_POINT('Ctrl Pts',(30.4199450706296,0.856752956966088,35.6417681188669));
#34792=CARTESIAN_POINT('Ctrl Pts',(30.5405284008673,0.955292659882133,35.5971805278559));
#34793=CARTESIAN_POINT('Ctrl Pts',(30.6877287941394,1.13847380954807,35.5425226152298));
#34794=CARTESIAN_POINT('Ctrl Pts',(30.7342206529605,1.21379195435447,35.525203642034));
#34795=CARTESIAN_POINT('Ctrl Pts',(30.7885863901995,1.3617131947964,35.5049304586299));
#34796=CARTESIAN_POINT('Ctrl Pts',(30.8017856625229,1.42978275763078,35.5));
#34797=CARTESIAN_POINT('Ctrl Pts',(30.8017856625229,1.5,35.5));
#34798=CARTESIAN_POINT('Origin',(53.2,1.5,0.));
#34799=CARTESIAN_POINT('',(58.,1.5,9.8974744253269));
#34800=CARTESIAN_POINT('Ctrl Pts',(59.5,0.,7.11055553385247));
#34801=CARTESIAN_POINT('Ctrl Pts',(59.4982621111229,-1.43714039392157E-18,
7.11441720740624));
#34802=CARTESIAN_POINT('Ctrl Pts',(59.4965230425191,3.02025636744488E-6,
7.11827835650607));
#34803=CARTESIAN_POINT('Ctrl Pts',(59.2998658347014,0.000687024107797401,
7.55454952423938));
#34804=CARTESIAN_POINT('Ctrl Pts',(59.0848279111169,0.0390861404131368,
7.99027457435745));
#34805=CARTESIAN_POINT('Ctrl Pts',(58.6790205873002,0.227280698650583,8.75389357006309));
#34806=CARTESIAN_POINT('Ctrl Pts',(58.5106474320198,0.353869330585071,9.04860693524593));
#34807=CARTESIAN_POINT('Ctrl Pts',(58.2889293801926,0.605541836240555,9.42608315641631));
#34808=CARTESIAN_POINT('Ctrl Pts',(58.2055841166437,0.725339698576898,9.56428617469307));
#34809=CARTESIAN_POINT('Ctrl Pts',(58.0942335303233,0.966223567273987,9.74614959515893));
#34810=CARTESIAN_POINT('Ctrl Pts',(58.0567637695508,1.07370986494963,9.80652098494185));
#34811=CARTESIAN_POINT('Ctrl Pts',(58.01124521301,1.29080573116058,9.87956234691206));
#34812=CARTESIAN_POINT('Ctrl Pts',(58.,1.3939909411326,9.89747442532689));
#34813=CARTESIAN_POINT('Ctrl Pts',(58.,1.5,9.89747442532689));
#34814=CARTESIAN_POINT('Origin',(53.2,1.5,0.));
#34815=CARTESIAN_POINT('Origin',(36.,1.5,13.5));
#34816=CARTESIAN_POINT('',(36.,1.5,35.5));
#34817=CARTESIAN_POINT('Origin',(36.,1.5,37.));
#34818=CARTESIAN_POINT('',(58.,1.5,13.5));
#34819=CARTESIAN_POINT('Origin',(36.,1.5,13.5));
#34820=CARTESIAN_POINT('Origin',(59.5,1.5,13.5));
#34821=CARTESIAN_POINT('Origin',(59.5,1.5,-1.5));
#34822=CARTESIAN_POINT('',(58.,1.5,-1.5));
#34823=CARTESIAN_POINT('Origin',(-18.,1.5,37.));
#34824=CARTESIAN_POINT('',(-18.,1.5,35.5));
#34825=CARTESIAN_POINT('Origin',(53.2,4.,0.));
#34826=CARTESIAN_POINT('',(58.,4.,9.8974744253269));
#34827=CARTESIAN_POINT('',(58.,4.,9.8974744253269));
#34828=CARTESIAN_POINT('',(46.2240601503759,4.,8.50507279301165));
#34829=CARTESIAN_POINT('Origin',(53.2,4.,0.));
#34830=CARTESIAN_POINT('',(46.2240601503759,4.,8.50507279301165));
#34831=CARTESIAN_POINT('Origin',(58.,0.,13.5));
#34832=CARTESIAN_POINT('',(58.,4.,13.5));
#34833=CARTESIAN_POINT('',(58.,0.,13.5));
#34834=CARTESIAN_POINT('',(58.,4.,-46.5));
#34835=CARTESIAN_POINT('Origin',(36.,0.,13.5));
#34836=CARTESIAN_POINT('',(36.,4.,35.5));
#34837=CARTESIAN_POINT('',(36.,0.,35.5));
#34838=CARTESIAN_POINT('Origin',(36.,4.,13.5));
#34839=CARTESIAN_POINT('Origin',(0.,1.5,0.));
#34840=CARTESIAN_POINT('Ctrl Pts',(17.7974717305574,1.5,43.5000000000001));
#34841=CARTESIAN_POINT('Ctrl Pts',(17.7974717305574,1.3081363470698,43.5000000000001));
#34842=CARTESIAN_POINT('Ctrl Pts',(17.7902374021495,1.11830736311257,43.4631927808952));
#34843=CARTESIAN_POINT('Ctrl Pts',(17.7620064094937,0.761470147690042,43.3198100779987));
#34844=CARTESIAN_POINT('Ctrl Pts',(17.7411731135178,0.598404516851343,43.2140759917526));
#34845=CARTESIAN_POINT('Ctrl Pts',(17.6880641128075,0.318992028184976,42.9452704489042));
#34846=CARTESIAN_POINT('Ctrl Pts',(17.6560897895307,0.206345030833379,42.7837511882912));
#34847=CARTESIAN_POINT('Ctrl Pts',(17.6020279405521,0.0861702418769968,
42.5115766866022));
#34848=CARTESIAN_POINT('Ctrl Pts',(17.5824878665501,0.0544158735673595,
42.4133539775058));
#34849=CARTESIAN_POINT('Ctrl Pts',(17.5423727024711,0.0114992072454748,
42.2120624504891));
#34850=CARTESIAN_POINT('Ctrl Pts',(17.5218884486073,0.000464895865378814,
42.1094502117176));
#34851=CARTESIAN_POINT('Ctrl Pts',(17.5008757674563,4.79373185133258E-6,
42.00437891946));
#34852=CARTESIAN_POINT('Ctrl Pts',(17.500437891852,9.05593823628022E-17,
42.0021894592601));
#34853=CARTESIAN_POINT('Ctrl Pts',(17.5,0.,42.0000000000001));
#34854=CARTESIAN_POINT('Ctrl Pts',(-17.5,0.,42.));
#34855=CARTESIAN_POINT('Ctrl Pts',(-17.500437891852,1.3406571373437E-19,
42.0021894592601));
#34856=CARTESIAN_POINT('Ctrl Pts',(-17.5008757674563,4.79373185123263E-6,
42.0043789194599));
#34857=CARTESIAN_POINT('Ctrl Pts',(-17.5218884486073,0.000464895865378844,
42.1094502117176));
#34858=CARTESIAN_POINT('Ctrl Pts',(-17.5423727024711,0.0114992072454764,
42.2120624504891));
#34859=CARTESIAN_POINT('Ctrl Pts',(-17.5824878665501,0.0544158735673544,
42.4133539775058));
#34860=CARTESIAN_POINT('Ctrl Pts',(-17.6020279405521,0.0861702418769902,
42.5115766866022));
#34861=CARTESIAN_POINT('Ctrl Pts',(-17.6560897895307,0.206345030833382,
42.7837511882912));
#34862=CARTESIAN_POINT('Ctrl Pts',(-17.6880641128075,0.31899202818498,42.9452704489042));
#34863=CARTESIAN_POINT('Ctrl Pts',(-17.7411731135178,0.598404516851343,
43.2140759917526));
#34864=CARTESIAN_POINT('Ctrl Pts',(-17.7620064094937,0.761470147690042,
43.3198100779987));
#34865=CARTESIAN_POINT('Ctrl Pts',(-17.7902374021495,1.11830736311257,43.4631927808952));
#34866=CARTESIAN_POINT('Ctrl Pts',(-17.7974717305574,1.3081363470698,43.5000000000001));
#34867=CARTESIAN_POINT('Ctrl Pts',(-17.7974717305574,1.5,43.5000000000001));
#34868=CARTESIAN_POINT('Origin',(0.,1.5,0.));
#34869=CARTESIAN_POINT('',(31.0449275599944,1.5,-35.2875682471136));
#34870=CARTESIAN_POINT('Origin',(0.,1.5,0.));
#34871=CARTESIAN_POINT('Ctrl Pts',(31.0952102098472,0.,-33.2165305534069));
#34872=CARTESIAN_POINT('Ctrl Pts',(31.0951696964714,-1.0480047872591E-17,
-33.2189876968878));
#34873=CARTESIAN_POINT('Ctrl Pts',(31.0951291138549,3.1191448844996E-6,
-33.2214448410094));
#34874=CARTESIAN_POINT('Ctrl Pts',(31.0915518419005,0.000552123420194366,
-33.4376681173871));
#34875=CARTESIAN_POINT('Ctrl Pts',(31.0874603040868,0.0247093974684173,
-33.6525355816948));
#34876=CARTESIAN_POINT('Ctrl Pts',(31.0787526147422,0.120411269801602,-34.0599327360631));
#34877=CARTESIAN_POINT('Ctrl Pts',(31.0741165440007,0.190507175290616,-34.2551775861872));
#34878=CARTESIAN_POINT('Ctrl Pts',(31.0646128476165,0.385154103985276,-34.6252458975057));
#34879=CARTESIAN_POINT('Ctrl Pts',(31.0596930143797,0.513035438790037,-34.8006041636678));
#34880=CARTESIAN_POINT('Ctrl Pts',(31.0522277771702,0.791102236957407,-35.0542336624389));
#34881=CARTESIAN_POINT('Ctrl Pts',(31.04943124825,0.9284220413215,-35.1446849201549));
#34882=CARTESIAN_POINT('Ctrl Pts',(31.0458481634946,1.21416954975876,-35.2589883222484));
#34883=CARTESIAN_POINT('Ctrl Pts',(31.0449275599943,1.35551696906064,-35.2875682471137));
#34884=CARTESIAN_POINT('Ctrl Pts',(31.0449275599943,1.5,-35.2875682471137));
#34885=CARTESIAN_POINT('Origin',(0.,4.,0.));
#34886=CARTESIAN_POINT('',(31.0449275599944,4.,-35.2875682471136));
#34887=CARTESIAN_POINT('Origin',(0.,4.,0.));
#34888=CARTESIAN_POINT('',(31.0449275599944,4.,-35.2875682471136));
#34889=CARTESIAN_POINT('Origin',(-53.2,1.5,0.));
#34890=CARTESIAN_POINT('',(-58.,1.5,-9.8974744253269));
#34891=CARTESIAN_POINT('Ctrl Pts',(-58.,1.5,-9.89747442532689));
#34892=CARTESIAN_POINT('Ctrl Pts',(-58.,1.3939909411326,-9.89747442532689));
#34893=CARTESIAN_POINT('Ctrl Pts',(-58.01124521301,1.29080573116058,-9.87956234691206));
#34894=CARTESIAN_POINT('Ctrl Pts',(-58.0567637695508,1.07370986494962,-9.80652098494185));
#34895=CARTESIAN_POINT('Ctrl Pts',(-58.0942335303233,0.966223567273955,
-9.7461495951589));
#34896=CARTESIAN_POINT('Ctrl Pts',(-58.2055841166437,0.725339698576908,
-9.56428617469307));
#34897=CARTESIAN_POINT('Ctrl Pts',(-58.2889293801925,0.605541836240571,
-9.42608315641633));
#34898=CARTESIAN_POINT('Ctrl Pts',(-58.5106474320197,0.3538693305852,-9.04860693524612));
#34899=CARTESIAN_POINT('Ctrl Pts',(-58.6790205873,0.22728069865065,-8.75389357006336));
#34900=CARTESIAN_POINT('Ctrl Pts',(-59.0848279111169,0.0390861404131358,
-7.99027457435745));
#34901=CARTESIAN_POINT('Ctrl Pts',(-59.2998658347014,0.000687024107797407,
-7.55454952423938));
#34902=CARTESIAN_POINT('Ctrl Pts',(-59.4965230425191,3.02025636744469E-6,
-7.11827835650607));
#34903=CARTESIAN_POINT('Ctrl Pts',(-59.4982621111229,-1.43714039392162E-18,
-7.11441720740624));
#34904=CARTESIAN_POINT('Ctrl Pts',(-59.5,0.,-7.11055553385247));
#34905=CARTESIAN_POINT('',(-46.2240601503759,1.5,-8.50507279301165));
#34906=CARTESIAN_POINT('Origin',(-53.2,1.5,0.));
#34907=CARTESIAN_POINT('Ctrl Pts',(-45.209022556391,0.,-5.13753632549022));
#34908=CARTESIAN_POINT('Ctrl Pts',(-45.2101706901698,-1.40306831947151E-18,
-5.1424595478439));
#34909=CARTESIAN_POINT('Ctrl Pts',(-45.2113202904361,2.87874308667369E-6,
-5.14738243736215));
#34910=CARTESIAN_POINT('Ctrl Pts',(-45.3805806080453,0.000852747691942822,
-5.87122802568613));
#34911=CARTESIAN_POINT('Ctrl Pts',(-45.5407068116734,0.0644575554238702,
-6.42770683878517));
#34912=CARTESIAN_POINT('Ctrl Pts',(-45.7992896021911,0.262676028338764,
-7.2772849093325));
#34913=CARTESIAN_POINT('Ctrl Pts',(-45.9058399421765,0.391768785578303,
-7.59761029794935));
#34914=CARTESIAN_POINT('Ctrl Pts',(-46.0437392091658,0.637700968927232,
-8.001083222404));
#34915=CARTESIAN_POINT('Ctrl Pts',(-46.095986299131,0.754435257863824,-8.14964878644436));
#34916=CARTESIAN_POINT('Ctrl Pts',(-46.165500553065,0.987918955923379,-8.34412682404563));
#34917=CARTESIAN_POINT('Ctrl Pts',(-46.188816675386,1.09129381988883,-8.40843236441881));
#34918=CARTESIAN_POINT('Ctrl Pts',(-46.2170785613611,1.2996923399296,-8.48604609926933));
#34919=CARTESIAN_POINT('Ctrl Pts',(-46.2240601503759,1.39848091468841,-8.50507279301164));
#34920=CARTESIAN_POINT('Ctrl Pts',(-46.2240601503759,1.5,-8.50507279301164));
#34921=CARTESIAN_POINT('Origin',(-53.2,4.,0.));
#34922=CARTESIAN_POINT('',(-58.,4.,-9.8974744253269));
#34923=CARTESIAN_POINT('',(-58.,4.,-9.8974744253269));
#34924=CARTESIAN_POINT('',(-46.2240601503759,4.,-8.50507279301165));
#34925=CARTESIAN_POINT('Origin',(-53.2,4.,0.));
#34926=CARTESIAN_POINT('',(-46.2240601503759,4.,-8.50507279301165));
#34927=CARTESIAN_POINT('Origin',(59.5,1.5,-1.5));
#34928=CARTESIAN_POINT('',(58.,1.5,-9.8974744253269));
#34929=CARTESIAN_POINT('',(58.,1.5,-46.5));
#34930=CARTESIAN_POINT('',(58.,1.5,-1.5));
#34931=CARTESIAN_POINT('Origin',(59.5,1.5,-46.5));
#34932=CARTESIAN_POINT('Ctrl Pts',(59.5,0.,-7.11055553385247));
#34933=CARTESIAN_POINT('Ctrl Pts',(59.4982621111222,-1.4371403945548E-18,
-7.11441720740794));
#34934=CARTESIAN_POINT('Ctrl Pts',(59.4965230425199,3.02025636478306E-6,
-7.11827835650437));
#34935=CARTESIAN_POINT('Ctrl Pts',(59.2998658346704,0.000687024107904035,
-7.55454952430768));
#34936=CARTESIAN_POINT('Ctrl Pts',(59.0848279111138,0.0390861404145931,
-7.99027457436337));
#34937=CARTESIAN_POINT('Ctrl Pts',(58.6790205873,0.22728069865069,-8.75389357006352));
#34938=CARTESIAN_POINT('Ctrl Pts',(58.5106474320196,0.353869330585278,-9.04860693524623));
#34939=CARTESIAN_POINT('Ctrl Pts',(58.2889293801926,0.60554183624056,-9.42608315641631));
#34940=CARTESIAN_POINT('Ctrl Pts',(58.2055841166437,0.725339698576902,-9.56428617469306));
#34941=CARTESIAN_POINT('Ctrl Pts',(58.0942335303233,0.966223567273979,-9.74614959515892));
#34942=CARTESIAN_POINT('Ctrl Pts',(58.0567637695508,1.07370986494963,-9.80652098494185));
#34943=CARTESIAN_POINT('Ctrl Pts',(58.01124521301,1.29080573116054,-9.87956234691204));
#34944=CARTESIAN_POINT('Ctrl Pts',(58.,1.39399094113258,-9.89747442532689));
#34945=CARTESIAN_POINT('Ctrl Pts',(58.,1.5,-9.89747442532689));
#34946=CARTESIAN_POINT('Origin',(53.2,1.5,0.));
#34947=CARTESIAN_POINT('',(46.2240601503759,1.5,-8.50507279301165));
#34948=CARTESIAN_POINT('Ctrl Pts',(45.209022556391,0.,-5.13753632549022));
#34949=CARTESIAN_POINT('Ctrl Pts',(45.2101706901698,-1.40306831936872E-18,
-5.14245954784354));
#34950=CARTESIAN_POINT('Ctrl Pts',(45.2113202904362,2.87874308709708E-6,
-5.14738243736251));
#34951=CARTESIAN_POINT('Ctrl Pts',(45.3805806079222,0.000852747691324604,
-5.87122802515958));
#34952=CARTESIAN_POINT('Ctrl Pts',(45.5407068115586,0.0644575553358579,
-6.42770683840794));
#34953=CARTESIAN_POINT('Ctrl Pts',(45.799289602191,0.26267602833871,-7.27728490933226));
#34954=CARTESIAN_POINT('Ctrl Pts',(45.9058399421765,0.391768785578204,-7.59761029794919));
#34955=CARTESIAN_POINT('Ctrl Pts',(46.0437392091658,0.637700968927248,-8.00108322240403));
#34956=CARTESIAN_POINT('Ctrl Pts',(46.095986299131,0.754435257863832,-8.14964878644437));
#34957=CARTESIAN_POINT('Ctrl Pts',(46.165500553065,0.98791895592338,-8.34412682404562));
#34958=CARTESIAN_POINT('Ctrl Pts',(46.188816675386,1.09129381988883,-8.40843236441881));
#34959=CARTESIAN_POINT('Ctrl Pts',(46.2170785613611,1.29969233992958,-8.48604609926932));
#34960=CARTESIAN_POINT('Ctrl Pts',(46.2240601503759,1.39848091468841,-8.50507279301164));
#34961=CARTESIAN_POINT('Ctrl Pts',(46.2240601503759,1.5,-8.50507279301164));
#34962=CARTESIAN_POINT('Origin',(53.2,1.5,0.));
#34963=CARTESIAN_POINT('Origin',(0.,1.5,0.));
#34964=CARTESIAN_POINT('',(35.2875682471136,1.5,-31.0449275599944));
#34965=CARTESIAN_POINT('Ctrl Pts',(35.2875682471136,1.5,-31.0449275599943));
#34966=CARTESIAN_POINT('Ctrl Pts',(35.2875682471136,1.35551696906072,-31.0449275599943));
#34967=CARTESIAN_POINT('Ctrl Pts',(35.2589883222484,1.2141695497589,-31.0458481634946));
#34968=CARTESIAN_POINT('Ctrl Pts',(35.1446849201549,0.928422041321496,-31.04943124825));
#34969=CARTESIAN_POINT('Ctrl Pts',(35.0542336624389,0.791102236957392,-31.0522277771702));
#34970=CARTESIAN_POINT('Ctrl Pts',(34.8006041636678,0.513035438790074,-31.0596930143797));
#34971=CARTESIAN_POINT('Ctrl Pts',(34.6252458975058,0.385154103985321,-31.0646128476165));
#34972=CARTESIAN_POINT('Ctrl Pts',(34.2551775861873,0.190507175290631,-31.0741165440007));
#34973=CARTESIAN_POINT('Ctrl Pts',(34.0599327360632,0.120411269801612,-31.0787526147422));
#34974=CARTESIAN_POINT('Ctrl Pts',(33.6525355816955,0.0247093974685881,
-31.0874603040868));
#34975=CARTESIAN_POINT('Ctrl Pts',(33.4376681173913,0.000552123420203993,
-31.0915518418999));
#34976=CARTESIAN_POINT('Ctrl Pts',(33.2214448410094,3.11914488445421E-6,
-31.0951291138549));
#34977=CARTESIAN_POINT('Ctrl Pts',(33.2189876968878,1.08143054073223E-19,
-31.0951696964714));
#34978=CARTESIAN_POINT('Ctrl Pts',(33.2165305534069,0.,-31.0952102098472));
#34979=CARTESIAN_POINT('Origin',(0.,1.5,0.));
#34980=CARTESIAN_POINT('Origin',(36.,1.5,-46.5));
#34981=CARTESIAN_POINT('',(36.,1.5,-68.5));
#34982=CARTESIAN_POINT('Origin',(36.,1.5,-70.));
#34983=CARTESIAN_POINT('Origin',(36.,1.5,-46.5));
#34984=CARTESIAN_POINT('Origin',(18.,1.5,-70.));
#34985=CARTESIAN_POINT('',(-36.,1.5,-68.5));
#34986=CARTESIAN_POINT('Origin',(-36.,1.5,-70.));
#34987=CARTESIAN_POINT('',(18.,1.5,-68.5));
#34988=CARTESIAN_POINT('Origin',(-36.,1.5,-46.5));
#34989=CARTESIAN_POINT('',(-58.,1.5,-46.5));
#34990=CARTESIAN_POINT('Origin',(-59.5,1.5,-46.5));
#34991=CARTESIAN_POINT('Origin',(-36.,1.5,-46.5));
#34992=CARTESIAN_POINT('Origin',(-59.5,1.5,-31.5));
#34993=CARTESIAN_POINT('',(-58.,1.5,-31.5));
#34994=CARTESIAN_POINT('Origin',(-58.,0.,-46.5));
#34995=CARTESIAN_POINT('',(-58.,4.,-46.5));
#34996=CARTESIAN_POINT('',(-58.,0.,-46.5));
#34997=CARTESIAN_POINT('',(-58.,4.,13.5));
#34998=CARTESIAN_POINT('Origin',(-36.,0.,-46.5));
#34999=CARTESIAN_POINT('',(-36.,4.,-68.5));
#35000=CARTESIAN_POINT('',(-36.,0.,-68.5));
#35001=CARTESIAN_POINT('Origin',(-36.,4.,-46.5));
#35002=CARTESIAN_POINT('Origin',(36.,0.,-68.5));
#35003=CARTESIAN_POINT('',(36.,4.,-68.5));
#35004=CARTESIAN_POINT('',(36.,0.,-68.5));
#35005=CARTESIAN_POINT('',(-36.,4.,-68.5));
#35006=CARTESIAN_POINT('Origin',(36.,0.,-46.5));
#35007=CARTESIAN_POINT('',(58.,4.,-46.5));
#35008=CARTESIAN_POINT('',(58.,0.,-46.5));
#35009=CARTESIAN_POINT('Origin',(36.,4.,-46.5));
#35010=CARTESIAN_POINT('Origin',(58.,0.,13.5));
#35011=CARTESIAN_POINT('',(58.,4.,-9.8974744253269));
#35012=CARTESIAN_POINT('',(58.,4.,-9.8974744253269));
#35013=CARTESIAN_POINT('',(58.,4.,-46.5));
#35014=CARTESIAN_POINT('Origin',(53.2,4.,0.));
#35015=CARTESIAN_POINT('',(46.2240601503759,4.,-8.50507279301165));
#35016=CARTESIAN_POINT('',(46.2240601503759,4.,-8.50507279301165));
#35017=CARTESIAN_POINT('Origin',(53.2,4.,0.));
#35018=CARTESIAN_POINT('Origin',(0.,4.,0.));
#35019=CARTESIAN_POINT('',(35.2875682471136,4.,-31.0449275599944));
#35020=CARTESIAN_POINT('',(35.2875682471136,4.,-31.0449275599944));
#35021=CARTESIAN_POINT('Origin',(0.,4.,0.));
#35022=CARTESIAN_POINT('Origin',(-64.5,1.5,-32.5));
#35023=CARTESIAN_POINT('',(-66.,1.5,15.5));
#35024=CARTESIAN_POINT('Origin',(-64.5,1.5,15.5));
#35025=CARTESIAN_POINT('',(-66.,1.5,-48.5));
#35026=CARTESIAN_POINT('',(-66.,1.5,-32.5));
#35027=CARTESIAN_POINT('Origin',(-64.5,1.5,-48.5));
#35028=CARTESIAN_POINT('Origin',(-38.,1.5,-48.5));
#35029=CARTESIAN_POINT('',(-38.,1.5,-76.5));
#35030=CARTESIAN_POINT('Origin',(-38.,1.5,-75.));
#35031=CARTESIAN_POINT('Origin',(-38.,1.5,-48.5));
#35032=CARTESIAN_POINT('Origin',(19.,1.5,-75.));
#35033=CARTESIAN_POINT('',(38.,1.5,-76.5));
#35034=CARTESIAN_POINT('Origin',(38.,1.5,-75.));
#35035=CARTESIAN_POINT('',(19.,1.5,-76.5));
#35036=CARTESIAN_POINT('Origin',(38.,1.5,-48.5));
#35037=CARTESIAN_POINT('',(66.,1.5,-48.5));
#35038=CARTESIAN_POINT('Origin',(64.5,1.5,-48.5));
#35039=CARTESIAN_POINT('Origin',(38.,1.5,-48.5));
#35040=CARTESIAN_POINT('Origin',(64.5,1.5,-0.500000000000003));
#35041=CARTESIAN_POINT('',(66.,1.5,15.5));
#35042=CARTESIAN_POINT('Origin',(64.5,1.5,15.5));
#35043=CARTESIAN_POINT('',(66.,1.5,-0.500000000000003));
#35044=CARTESIAN_POINT('Origin',(38.,1.5,15.5));
#35045=CARTESIAN_POINT('',(38.,1.5,43.5));
#35046=CARTESIAN_POINT('Origin',(38.,1.5,42.));
#35047=CARTESIAN_POINT('Origin',(38.,1.5,15.5));
#35048=CARTESIAN_POINT('Origin',(-19.,1.5,42.));
#35049=CARTESIAN_POINT('',(-19.,1.5,43.5));
#35050=CARTESIAN_POINT('Origin',(-38.,1.5,15.5));
#35051=CARTESIAN_POINT('',(-38.,1.5,43.5));
#35052=CARTESIAN_POINT('Origin',(-38.,1.5,42.));
#35053=CARTESIAN_POINT('Origin',(-38.,1.5,15.5));
#35054=CARTESIAN_POINT('Origin',(-19.,1.5,42.));
#35055=CARTESIAN_POINT('',(-19.,1.5,43.5));
#35056=CARTESIAN_POINT('Origin',(38.,0.,-48.5));
#35057=CARTESIAN_POINT('',(38.,16.5,-76.5));
#35058=CARTESIAN_POINT('',(38.,0.,-76.5));
#35059=CARTESIAN_POINT('',(66.,16.5,-48.5));
#35060=CARTESIAN_POINT('Origin',(38.,16.5,-48.5));
#35061=CARTESIAN_POINT('',(66.,0.,-48.5));
#35062=CARTESIAN_POINT('Origin',(38.,0.,-76.5));
#35063=CARTESIAN_POINT('',(-38.,16.5,-76.5));
#35064=CARTESIAN_POINT('',(-38.,0.,-76.5));
#35065=CARTESIAN_POINT('',(19.,16.5,-76.5));
#35066=CARTESIAN_POINT('Origin',(-38.,0.,-48.5));
#35067=CARTESIAN_POINT('',(-66.,16.5,-48.5));
#35068=CARTESIAN_POINT('',(-66.,0.,-48.5));
#35069=CARTESIAN_POINT('Origin',(-38.,16.5,-48.5));
#35070=CARTESIAN_POINT('Origin',(-66.,0.,-48.5));
#35071=CARTESIAN_POINT('',(-66.,16.5,15.5));
#35072=CARTESIAN_POINT('',(-66.,0.,15.5));
#35073=CARTESIAN_POINT('',(-66.,16.5,-32.5));
#35074=CARTESIAN_POINT('Origin',(-38.,0.,15.5));
#35075=CARTESIAN_POINT('',(-38.,16.5,43.5));
#35076=CARTESIAN_POINT('',(-38.,0.,43.5));
#35077=CARTESIAN_POINT('Origin',(-38.,16.5,15.5));
#35078=CARTESIAN_POINT('Origin',(28.5201839509359,1.5,-26.3988636073762));
#35079=CARTESIAN_POINT('',(29.5808441227157,1.5,-25.3382034355964));
#35080=CARTESIAN_POINT('Origin',(48.7903679018718,4.,-44.5477272147525));
#35081=CARTESIAN_POINT('',(29.5808441227157,4.,-25.3382034355964));
#35082=CARTESIAN_POINT('Origin',(18.6206890143242,1.5,-20.7420093578839));
#35083=CARTESIAN_POINT('',(17.5600288425444,1.5,-21.8026695296637));
#35084=CARTESIAN_POINT('Origin',(28.9913780286485,4.,-33.2340187157677));
#35085=CARTESIAN_POINT('',(17.5600288425444,4.,-21.8026695296637));
#35086=CARTESIAN_POINT('Origin',(0.,1.5,0.));
#35087=CARTESIAN_POINT('',(-3.,1.5,-46.9041575982343));
#35088=CARTESIAN_POINT('Origin',(0.,1.5,0.));
#35089=CARTESIAN_POINT('Ctrl Pts',(-1.49999999999999,0.,-45.4752680036083));
#35090=CARTESIAN_POINT('Ctrl Pts',(-1.50176867612921,1.08300178019032E-19,
-45.4769793019272));
#35091=CARTESIAN_POINT('Ctrl Pts',(-1.50353740181665,3.12821524582445E-6,
-45.4786905515984));
#35092=CARTESIAN_POINT('Ctrl Pts',(-1.6589485445968,0.000552890155855249,
-45.6290430115593));
#35093=CARTESIAN_POINT('Ctrl Pts',(-1.81376170731676,0.0247066439280583,
-45.7780704433202));
#35094=CARTESIAN_POINT('Ctrl Pts',(-2.10792859962105,0.120380195566533,
-46.059925664155));
#35095=CARTESIAN_POINT('Ctrl Pts',(-2.24921701551043,0.190439066398323,
-46.1946602843644));
#35096=CARTESIAN_POINT('Ctrl Pts',(-2.51762496582942,0.385035588736779,
-46.4496283712152));
#35097=CARTESIAN_POINT('Ctrl Pts',(-2.64514766490965,0.512937531198891,
-46.5701910337406));
#35098=CARTESIAN_POINT('Ctrl Pts',(-2.82982150540341,0.791053413169234,
-46.7443046032146));
#35099=CARTESIAN_POINT('Ctrl Pts',(-2.89577102625226,0.928389940435116,
-46.8062984441602));
#35100=CARTESIAN_POINT('Ctrl Pts',(-2.97913882256007,1.21416179467569,-46.8845984232444));
#35101=CARTESIAN_POINT('Ctrl Pts',(-3.,1.35551296703019,-46.9041575982343));
#35102=CARTESIAN_POINT('Ctrl Pts',(-3.,1.5,-46.9041575982343));
#35103=CARTESIAN_POINT('Origin',(-20.7420093578839,1.5,-18.6206890143242));
#35104=CARTESIAN_POINT('',(-35.2875682471136,1.5,-31.0449275599944));
#35105=CARTESIAN_POINT('Ctrl Pts',(-33.2165305534069,0.,-31.0952102098472));
#35106=CARTESIAN_POINT('Ctrl Pts',(-33.2190692967299,1.11734401589879E-19,
-31.0951683510534));
#35107=CARTESIAN_POINT('Ctrl Pts',(-33.2216080407998,3.32975363937025E-6,
-31.0951264183426));
#35108=CARTESIAN_POINT('Ctrl Pts',(-33.4374895579293,0.000569671234467164,
-31.0915543966548));
#35109=CARTESIAN_POINT('Ctrl Pts',(-33.6519250591449,0.0246506601297224,
-31.0874717825085));
#35110=CARTESIAN_POINT('Ctrl Pts',(-34.0573511387189,0.119724494999935,
-31.0788092838542));
#35111=CARTESIAN_POINT('Ctrl Pts',(-34.2510845845319,0.18899207660016,-31.0742145020815));
#35112=CARTESIAN_POINT('Ctrl Pts',(-34.6214706148708,0.382511576258843,
-31.0647171688647));
#35113=CARTESIAN_POINT('Ctrl Pts',(-34.7982799030232,0.510857073213111,
-31.0597601262273));
#35114=CARTESIAN_POINT('Ctrl Pts',(-35.0535067624131,0.790024881159229,
-31.0522501584557));
#35115=CARTESIAN_POINT('Ctrl Pts',(-35.1443641805612,0.927714535375577,
-31.0494412598632));
#35116=CARTESIAN_POINT('Ctrl Pts',(-35.2589537310755,1.21399986481142,-31.0458492854634));
#35117=CARTESIAN_POINT('Ctrl Pts',(-35.2875682471136,1.35542940125323,-31.0449275599943));
#35118=CARTESIAN_POINT('Ctrl Pts',(-35.2875682471136,1.5,-31.0449275599943));
#35119=CARTESIAN_POINT('',(-21.8026695296637,1.5,-17.5600288425444));
#35120=CARTESIAN_POINT('Origin',(0.,1.5,0.));
#35121=CARTESIAN_POINT('Origin',(0.,1.5,0.));
#35122=CARTESIAN_POINT('Origin',(0.,4.,0.));
#35123=CARTESIAN_POINT('',(-3.,4.,-46.9041575982343));
#35124=CARTESIAN_POINT('Origin',(0.,4.,0.));
#35125=CARTESIAN_POINT('',(-3.,4.,-46.9041575982343));
#35126=CARTESIAN_POINT('Origin',(-33.2340187157677,4.,-28.9913780286484));
#35127=CARTESIAN_POINT('',(-35.2875682471136,4.,-31.0449275599944));
#35128=CARTESIAN_POINT('',(-35.2875682471136,4.,-31.0449275599944));
#35129=CARTESIAN_POINT('',(-21.8026695296637,4.,-17.5600288425444));
#35130=CARTESIAN_POINT('Origin',(0.,4.,0.));
#35131=CARTESIAN_POINT('Origin',(0.,4.,0.));
#35132=CARTESIAN_POINT('Origin',(38.,16.5,-48.5));
#35133=CARTESIAN_POINT('Origin',(64.5,16.5,-48.5));
#35134=CARTESIAN_POINT('Origin',(38.,16.5,-75.));
#35135=CARTESIAN_POINT('Origin',(19.,16.5,-75.));
#35136=CARTESIAN_POINT('Origin',(-38.,16.5,-75.));
#35137=CARTESIAN_POINT('Origin',(-38.,16.5,-48.5));
#35138=CARTESIAN_POINT('Origin',(-64.5,16.5,-48.5));
#35139=CARTESIAN_POINT('Origin',(-64.5,16.5,-32.5));
#35140=CARTESIAN_POINT('Origin',(-64.5,16.5,15.5));
#35141=CARTESIAN_POINT('Origin',(-38.,16.5,15.5));
#35142=CARTESIAN_POINT('Origin',(-38.,16.5,42.));
#35143=CARTESIAN_POINT('Origin',(-19.,16.5,42.));
#35144=CARTESIAN_POINT('',(38.,16.5,43.5));
#35145=CARTESIAN_POINT('Origin',(38.,16.5,42.));
#35146=CARTESIAN_POINT('',(-19.,16.5,43.5));
#35147=CARTESIAN_POINT('Origin',(38.,16.5,15.5));
#35148=CARTESIAN_POINT('',(66.,16.5,15.5));
#35149=CARTESIAN_POINT('Origin',(64.5,16.5,15.5));
#35150=CARTESIAN_POINT('Origin',(38.,16.5,15.5));
#35151=CARTESIAN_POINT('Origin',(64.5,16.5,-0.500000000000003));
#35152=CARTESIAN_POINT('',(66.,16.5,-0.500000000000003));
#35153=CARTESIAN_POINT('Origin',(0.,-4.5,0.));
#35154=CARTESIAN_POINT('',(9.86076131526265E-31,-4.5,-41.28));
#35155=CARTESIAN_POINT('Origin',(0.,-4.5,0.));
#35156=CARTESIAN_POINT('',(-9.74328993401634E-15,-6.,-39.78));
#35157=CARTESIAN_POINT('Origin',(9.8065271280287E-31,-4.5,-39.78));
#35158=CARTESIAN_POINT('Origin',(0.,-6.,0.));
#35159=CARTESIAN_POINT('Origin',(0.,-2.7,0.));
#35160=CARTESIAN_POINT('Origin',(0.,-1.8,0.));
#35161=CARTESIAN_POINT('Ctrl Pts',(30.8986928114497,0.551098954354967,27.3735124261331));
#35162=CARTESIAN_POINT('Ctrl Pts',(30.8641827118076,0.506664989272846,27.4124667609344));
#35163=CARTESIAN_POINT('Ctrl Pts',(30.8279866393545,0.464974641768682,27.4531744708043));
#35164=CARTESIAN_POINT('Ctrl Pts',(30.65814747972,0.288491142640607,27.6433707222812));
#35165=CARTESIAN_POINT('Ctrl Pts',(30.5070255439578,0.182453844116018,27.810330268993));
#35166=CARTESIAN_POINT('Ctrl Pts',(30.1879066118572,0.0382329615783753,
28.1564350499007));
#35167=CARTESIAN_POINT('Ctrl Pts',(30.0175971548222,3.00801135180405E-15,
28.3380263942472));
#35168=CARTESIAN_POINT('Ctrl Pts',(29.8463073008423,1.11022302462516E-15,
28.5172989692869));
#35169=CARTESIAN_POINT('Ctrl Pts',(-29.8463073008423,1.14491749414469E-15,
28.5172989692869));
#35170=CARTESIAN_POINT('Ctrl Pts',(-30.0635571076826,3.52780524293222E-15,
28.2899245428733));
#35171=CARTESIAN_POINT('Ctrl Pts',(-30.2801233439677,0.0616272685536241,
28.0577630238579));
#35172=CARTESIAN_POINT('Ctrl Pts',(-30.6381675045497,0.272254431305175,
27.665825911273));
#35173=CARTESIAN_POINT('Ctrl Pts',(-30.7814255694024,0.400109864424864,
27.5058814269562));
#35174=CARTESIAN_POINT('Ctrl Pts',(-30.898692811445,0.551098954348924,27.3735124261384));
#35175=CARTESIAN_POINT('Origin',(0.,-1.8,0.));
#35176=CARTESIAN_POINT('Ctrl Pts',(-35.7247978384162,0.551098954354972,
20.6827759114751));
#35177=CARTESIAN_POINT('Ctrl Pts',(-35.7508728501454,0.506664989272856,
20.6377372509662));
#35178=CARTESIAN_POINT('Ctrl Pts',(-35.7780796730643,0.464974641768688,
20.590545492252));
#35179=CARTESIAN_POINT('Ctrl Pts',(-35.9049685855587,0.288491142640602,
20.3693687346412));
#35180=CARTESIAN_POINT('Ctrl Pts',(-36.0157138907406,0.182453844116013,
20.1732850609533));
#35181=CARTESIAN_POINT('Ctrl Pts',(-36.2434429291201,0.0382329615783755,
19.7612597009681));
#35182=CARTESIAN_POINT('Ctrl Pts',(-36.3620181378251,3.00801135180405E-15,
19.5423518496295));
#35183=CARTESIAN_POINT('Ctrl Pts',(-36.4780836837786,1.11022302462516E-15,
19.3232453474888));
#35184=CARTESIAN_POINT('',(-5.05534198688027E-15,-2.7,-41.28));
#35185=CARTESIAN_POINT('Ctrl Pts',(36.4780836837786,1.21430643318376E-15,
19.3232453474888));
#35186=CARTESIAN_POINT('Ctrl Pts',(36.330875796952,2.8116267922611E-15,
19.601141814568));
#35187=CARTESIAN_POINT('Ctrl Pts',(36.1789096837638,0.0616272685536261,
19.8799001436861));
#35188=CARTESIAN_POINT('Ctrl Pts',(35.9199721561489,0.272254431305173,20.3433240079195));
#35189=CARTESIAN_POINT('Ctrl Pts',(35.8134021815952,0.400109864424854,20.5297320327797));
#35190=CARTESIAN_POINT('Ctrl Pts',(35.7247978384197,0.551098954348926,20.682775911469));
#35191=CARTESIAN_POINT('Origin',(0.,-6.,40.78));
#35192=CARTESIAN_POINT('',(-1.75124492278072E-15,-6.,-14.3));
#35193=CARTESIAN_POINT('Origin',(0.,-6.,0.));
#35194=CARTESIAN_POINT('Origin',(-1.5,1.5,-30.25));
#35195=CARTESIAN_POINT('',(-3.,1.5,-30.25));
#35196=CARTESIAN_POINT('Origin',(-3.,4.,-44.));
#35197=CARTESIAN_POINT('',(-3.,4.,-30.25));
#35198=CARTESIAN_POINT('Origin',(30.5,1.5,22.));
#35199=CARTESIAN_POINT('Origin',(0.,-1.8,0.));
#35200=CARTESIAN_POINT('Origin',(0.,-0.3,0.));
#35201=CARTESIAN_POINT('Origin',(30.5,-0.3,22.));
#35202=CARTESIAN_POINT('Origin',(-30.5,1.5,22.));
#35203=CARTESIAN_POINT('Origin',(0.,-1.8,0.));
#35204=CARTESIAN_POINT('Origin',(0.,-0.3,0.));
#35205=CARTESIAN_POINT('Origin',(-30.5,-0.3,22.));
#35206=CARTESIAN_POINT('Origin',(26.05,16.5,-24.75));
#35207=CARTESIAN_POINT('',(24.55,16.5,-33.));
#35208=CARTESIAN_POINT('Origin',(26.05,16.5,-33.));
#35209=CARTESIAN_POINT('',(24.55,16.5,3.00650789190675E-15));
#35210=CARTESIAN_POINT('',(24.55,16.5,-24.75));
#35211=CARTESIAN_POINT('Origin',(26.05,16.5,4.44089209850063E-15));
#35212=CARTESIAN_POINT('Origin',(0.,16.5,0.));
#35213=CARTESIAN_POINT('',(-24.55,16.5,0.));
#35214=CARTESIAN_POINT('Origin',(-26.05,16.5,0.));
#35215=CARTESIAN_POINT('Origin',(0.,16.5,0.));
#35216=CARTESIAN_POINT('Origin',(-26.05,16.5,-8.25));
#35217=CARTESIAN_POINT('',(-24.55,16.5,-33.));
#35218=CARTESIAN_POINT('Origin',(-26.05,16.5,-33.));
#35219=CARTESIAN_POINT('',(-24.55,16.5,-8.25));
#35220=CARTESIAN_POINT('Origin',(0.,16.5,-33.));
#35221=CARTESIAN_POINT('Origin',(0.,16.5,-33.));
#35222=CARTESIAN_POINT('Origin',(0.,18.,0.));
#35223=CARTESIAN_POINT('',(24.55,15.95,3.00650789190675E-15));
#35224=CARTESIAN_POINT('',(24.55,18.,3.00650789190675E-15));
#35225=CARTESIAN_POINT('',(-24.55,15.95,0.));
#35226=CARTESIAN_POINT('Origin',(0.,15.95,0.));
#35227=CARTESIAN_POINT('',(-24.55,18.,0.));
#35228=CARTESIAN_POINT('Origin',(24.55,18.,-33.));
#35229=CARTESIAN_POINT('',(24.55,15.95,-33.));
#35230=CARTESIAN_POINT('',(24.55,18.,-33.));
#35231=CARTESIAN_POINT('',(24.55,15.95,0.));
#35232=CARTESIAN_POINT('Origin',(-20.95,16.5,-24.75));
#35233=CARTESIAN_POINT('',(-22.45,16.5,-33.));
#35234=CARTESIAN_POINT('Origin',(-20.95,16.5,-33.));
#35235=CARTESIAN_POINT('',(-22.45,16.5,0.));
#35236=CARTESIAN_POINT('',(-22.45,16.5,-24.75));
#35237=CARTESIAN_POINT('Origin',(-20.95,16.5,0.));
#35238=CARTESIAN_POINT('Origin',(0.,16.5,0.));
#35239=CARTESIAN_POINT('',(22.45,16.5,2.74933206408581E-15));
#35240=CARTESIAN_POINT('Origin',(20.95,16.5,2.5656350442137E-15));
#35241=CARTESIAN_POINT('Origin',(0.,16.5,0.));
#35242=CARTESIAN_POINT('Origin',(20.95,16.5,-8.25));
#35243=CARTESIAN_POINT('',(22.45,16.5,-33.));
#35244=CARTESIAN_POINT('Origin',(20.95,16.5,-33.));
#35245=CARTESIAN_POINT('',(22.45,16.5,-8.25));
#35246=CARTESIAN_POINT('Origin',(0.,16.5,-33.));
#35247=CARTESIAN_POINT('Origin',(0.,16.5,-33.));
#35248=CARTESIAN_POINT('Origin',(0.,18.,0.));
#35249=CARTESIAN_POINT('',(-22.45,15.95,0.));
#35250=CARTESIAN_POINT('',(-22.45,18.,0.));
#35251=CARTESIAN_POINT('',(22.45,15.95,2.74933206408581E-15));
#35252=CARTESIAN_POINT('Origin',(0.,15.95,0.));
#35253=CARTESIAN_POINT('',(22.45,18.,2.74933206408581E-15));
#35254=CARTESIAN_POINT('Origin',(-22.45,18.,-33.));
#35255=CARTESIAN_POINT('',(-22.45,15.95,-33.));
#35256=CARTESIAN_POINT('',(-22.45,18.,-33.));
#35257=CARTESIAN_POINT('',(-22.45,15.95,-33.));
#35258=CARTESIAN_POINT('Origin',(0.,18.,-33.));
#35259=CARTESIAN_POINT('',(22.45,15.95,-33.));
#35260=CARTESIAN_POINT('',(22.45,18.,-33.));
#35261=CARTESIAN_POINT('Origin',(0.,15.95,-33.));
#35262=CARTESIAN_POINT('Origin',(22.45,18.,0.));
#35263=CARTESIAN_POINT('',(22.45,15.95,0.));
#35264=CARTESIAN_POINT('Origin',(0.,18.,-33.));
#35265=CARTESIAN_POINT('',(-24.55,15.95,-33.));
#35266=CARTESIAN_POINT('',(-24.55,18.,-33.));
#35267=CARTESIAN_POINT('Origin',(0.,15.95,-33.));
#35268=CARTESIAN_POINT('Origin',(-24.55,18.,0.));
#35269=CARTESIAN_POINT('',(-24.55,15.95,-33.));
#35270=CARTESIAN_POINT('Origin',(0.,15.95,-16.5));
#35271=CARTESIAN_POINT('Origin',(30.5,18.,-16.5));
#35272=CARTESIAN_POINT('',(26.49,9.9,-16.5));
#35273=CARTESIAN_POINT('',(26.49,18.,-16.5));
#35274=CARTESIAN_POINT('Origin',(30.5,9.9,-16.5));
#35275=CARTESIAN_POINT('Origin',(30.5,9.9,-16.5));
#35276=CARTESIAN_POINT('Origin',(-30.5,18.,-16.5));
#35277=CARTESIAN_POINT('',(-34.51,9.9,-16.5));
#35278=CARTESIAN_POINT('',(-34.51,18.,-16.5));
#35279=CARTESIAN_POINT('Origin',(-30.5,9.9,-16.5));
#35280=CARTESIAN_POINT('Origin',(-30.5,9.9,-16.5));
#35281=CARTESIAN_POINT('Origin',(0.,-5.5,14.7));
#35282=CARTESIAN_POINT('',(-1.80023079474661E-15,-5.5,-14.7));
#35283=CARTESIAN_POINT('Origin',(0.,-5.5,0.));
#35284=CARTESIAN_POINT('',(-1.75124492278072E-15,-5.5,-14.3));
#35285=CARTESIAN_POINT('Origin',(0.,-5.5,0.));
#35286=CARTESIAN_POINT('Origin',(0.,-4.85,0.));
#35287=CARTESIAN_POINT('',(-1.80023079474661E-15,-4.2,-14.7));
#35288=CARTESIAN_POINT('',(-1.80023079474661E-15,-4.85,-14.7));
#35289=CARTESIAN_POINT('Origin',(0.,-4.2,0.));
#35290=CARTESIAN_POINT('Origin',(0.,-4.2,14.2));
#35291=CARTESIAN_POINT('',(1.75124492278072E-15,-4.2,-14.3));
#35292=CARTESIAN_POINT('Origin',(0.,-4.2,0.));
#35293=CARTESIAN_POINT('Origin',(0.,-2.,0.));
#35294=CARTESIAN_POINT('',(-1.75124492278072E-15,-2.,-14.3));
#35295=CARTESIAN_POINT('Origin',(0.,-2.,0.));
#35296=CARTESIAN_POINT('',(-1.75124492278072E-15,-2.,-14.3));
#35297=CARTESIAN_POINT('Origin',(0.,4.,-16.5));
#35298=CARTESIAN_POINT('Origin',(0.,4.,0.));
#35299=CARTESIAN_POINT('',(30.8017856625229,4.,35.5));
#35300=CARTESIAN_POINT('Origin',(0.,4.,0.));
#35301=CARTESIAN_POINT('',(30.8017856625229,4.,35.5));
#35302=CARTESIAN_POINT('Origin',(-53.2,4.,0.));
#35303=CARTESIAN_POINT('',(-58.,4.,9.8974744253269));
#35304=CARTESIAN_POINT('Origin',(-53.2,4.,0.));
#35305=CARTESIAN_POINT('',(-58.,4.,9.8974744253269));
#35306=CARTESIAN_POINT('Origin',(0.,4.,0.));
#35307=CARTESIAN_POINT('',(-19.,4.,43.5));
#35308=CARTESIAN_POINT('Origin',(-38.,0.,43.5));
#35309=CARTESIAN_POINT('',(38.,0.,43.5));
#35310=CARTESIAN_POINT('Origin',(-58.,0.,-46.5));
#35311=CARTESIAN_POINT('',(-58.,4.,13.5));
#35312=CARTESIAN_POINT('Origin',(-36.,0.,35.5));
#35313=CARTESIAN_POINT('',(36.,4.,35.5));
#35314=CARTESIAN_POINT('Origin',(0.,4.,-16.5));
#35315=CARTESIAN_POINT('Origin',(0.,4.,-16.5));
#35316=CARTESIAN_POINT('Origin',(66.,0.,15.5));
#35317=CARTESIAN_POINT('',(66.,0.,15.5));
#35318=CARTESIAN_POINT('Origin',(38.,0.,15.5));
#46365=UNCERTAINTY_MEASURE_WITH_UNIT(LENGTH_MEASURE(0.01),#46396,
'DISTANCE_ACCURACY_VALUE',
'Maximum model space distance between geometric entities at asserted c
onnectivities');
#46379=UNCERTAINTY_MEASURE_WITH_UNIT(LENGTH_MEASURE(0.01),#46396,
'DISTANCE_ACCURACY_VALUE',
'Maximum model space distance between geometric entities at asserted c
onnectivities');
#46381=(
GEOMETRIC_REPRESENTATION_CONTEXT(3)
GLOBAL_UNCERTAINTY_ASSIGNED_CONTEXT((#46365))
GLOBAL_UNIT_ASSIGNED_CONTEXT((#46396,#46398,#46399))
REPRESENTATION_CONTEXT('','3D')
);
#46395=(
GEOMETRIC_REPRESENTATION_CONTEXT(3)
GLOBAL_UNCERTAINTY_ASSIGNED_CONTEXT((#46379))
GLOBAL_UNIT_ASSIGNED_CONTEXT((#46396,#46398,#46399))
REPRESENTATION_CONTEXT('','3D')
);
#46396=(
LENGTH_UNIT()
NAMED_UNIT(*)
SI_UNIT(.MILLI.,.METRE.)
);
#46398=(
NAMED_UNIT(*)
PLANE_ANGLE_UNIT()
SI_UNIT($,.RADIAN.)
);
#46399=(
NAMED_UNIT(*)
SI_UNIT($,.STERADIAN.)
SOLID_ANGLE_UNIT()
);
#46401=SHAPE_DEFINITION_REPRESENTATION(#46416,#46456);
#46416=PRODUCT_DEFINITION_SHAPE('',$,#46472);
#46456=SHAPE_REPRESENTATION('',(#25107),#46381);
#46470=PRODUCT_DEFINITION_CONTEXT('part definition',#46517,'design');
#46472=PRODUCT_DEFINITION('2026-10-26-00-50-38-164',
'01_Front_Flange_SAE_A',#46487,#46470);
#46487=PRODUCT_DEFINITION_FORMATION('',$,#46520);
#46517=APPLICATION_CONTEXT(
'Core Data for Automotive Mechanical Design Process');
#46518=PRODUCT_CONTEXT('part definition',#46517,'mechanical');
#46520=PRODUCT('2026-10-26-00-50-38-164','01_Front_Flange_SAE_A',$,(#46518));
#46583=COLOUR_RGB('Sky Blue',0.24,0.69,0.87);
#46584=FILL_AREA_STYLE_COLOUR('',#46583);
#46585=FILL_AREA_STYLE('',(#46584));
#46586=SURFACE_STYLE_FILL_AREA(#46585);
#46587=SURFACE_SIDE_STYLE('',(#46586));
#46588=SURFACE_STYLE_USAGE(.BOTH.,#46587);
#46589=PRESENTATION_STYLE_ASSIGNMENT((#46588));
ENDSEC;
END-ISO-10303-21;
